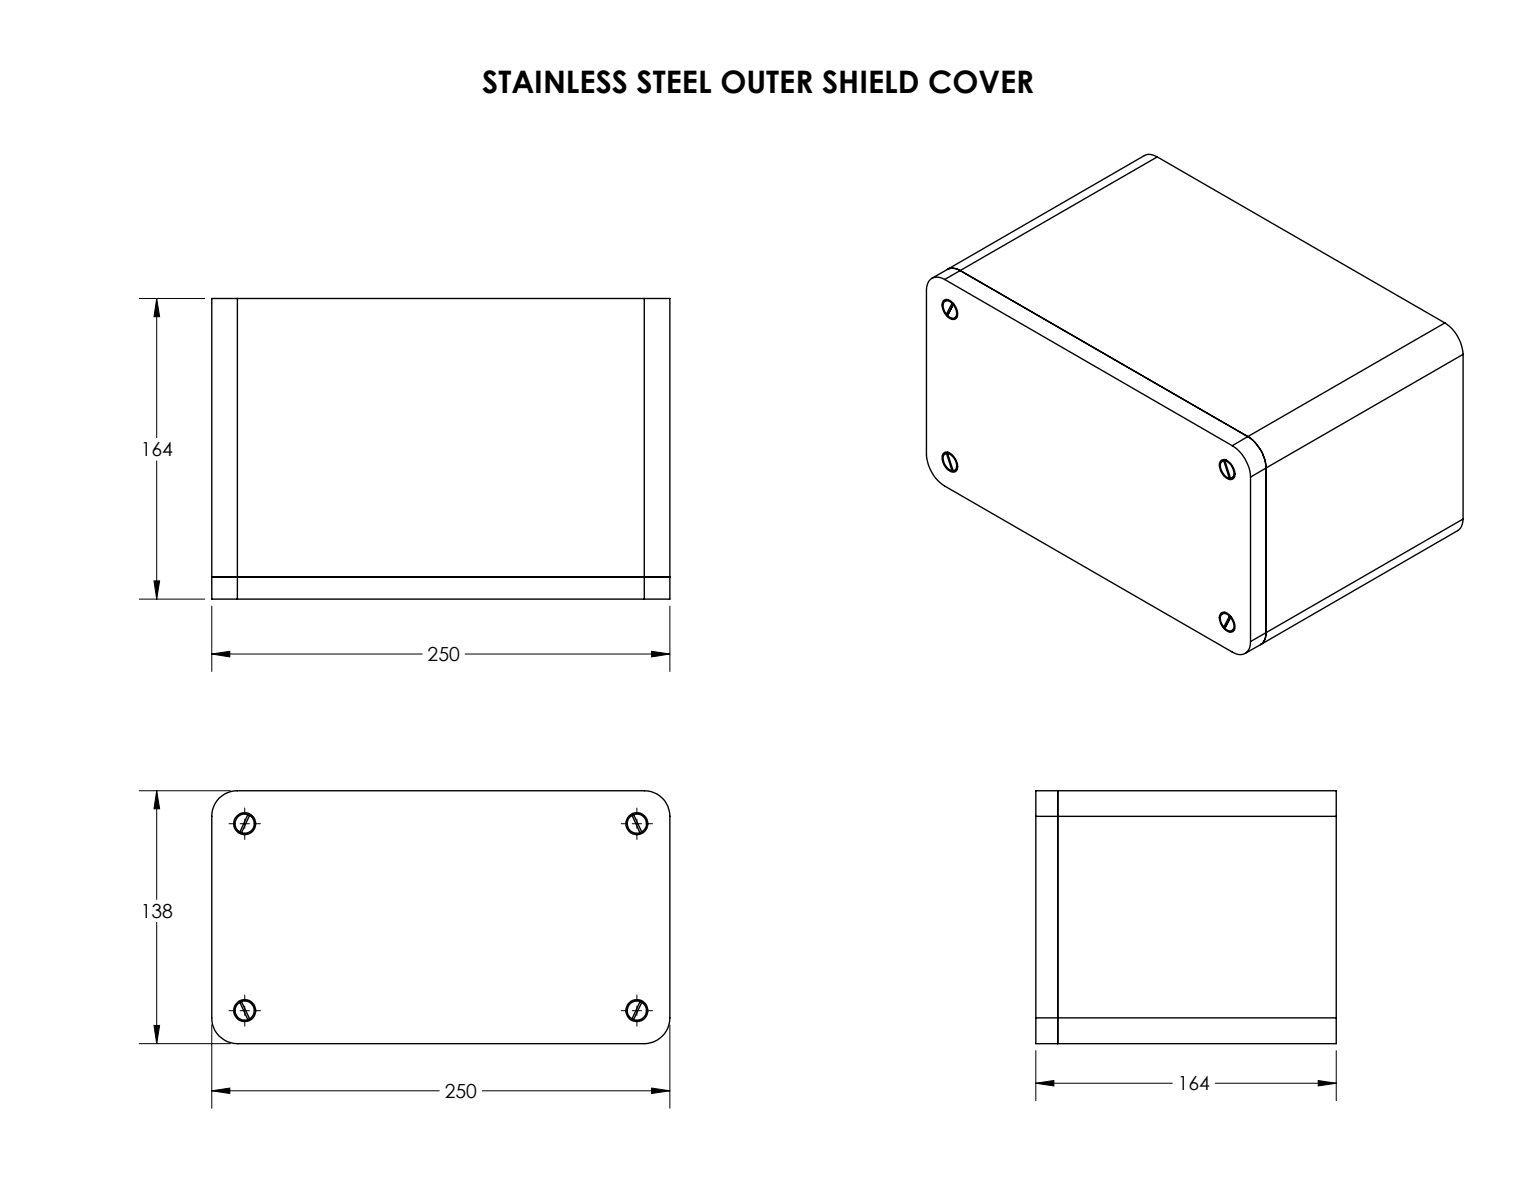
ISO-10303-21;
HEADER;
FILE_DESCRIPTION (('STEP AP214'),
    '1' );
FILE_NAME ('Stainless Steel Outer Shield Cover.step',
    '2026-10-28T18:30:06',
    ( '' ),
    ( '' ),
    'SwSTEP 2.0',
    'SolidWorks 2024',
    '' );
FILE_SCHEMA (( 'AUTOMOTIVE_DESIGN' ));
ENDSEC;

DATA;
#2=ORIENTED_EDGE ( 'NONE', *, *, #5398, .F. ) ;
#4=DIRECTION ( 'NONE',  ( 5.551115123125772841E-17, -1.848892746611743135E-31, -1.000000000000000000 ) ) ;
#6=CARTESIAN_POINT ( 'NONE',  ( -84.02857808274397655, 98.45434506795682239, 152.0000000000000853 ) ) ;
#9=ORIENTED_EDGE ( 'NONE', *, *, #3496, .F. ) ;
#10=DIRECTION ( 'NONE',  ( 0.4205749795070160557, -0.9072577839912276954, -5.551115123125780853E-17 ) ) ;
#13=EDGE_CURVE ( 'NONE', #832, #1072, #4200, .T. ) ;
#15=VECTOR ( 'NONE', #512, 1000.000000000000000 ) ;
#21=VECTOR ( 'NONE', #4832, 999.9999999999998863 ) ;
#23=CARTESIAN_POINT ( 'NONE',  ( -84.02857808274400497, -39.54565493204319182, -5.551115123125782702E-14 ) ) ;
#25=AXIS2_PLACEMENT_3D ( 'NONE', #1773, #1368, #5093 ) ;
#27=DIRECTION ( 'NONE',  ( -1.000000000000000000, 0.000000000000000000, -7.228014483236656373E-17 ) ) ;
#33=DIRECTION ( 'NONE',  ( 1.000000000000000000, 0.000000000000000000, 0.000000000000000000 ) ) ;
#41=DIRECTION ( 'NONE',  ( -1.000000000000000000, 0.000000000000000000, 0.000000000000000000 ) ) ;
#46=CYLINDRICAL_SURFACE ( 'NONE', #25, 6.000000000000032863 ) ;
#50=CARTESIAN_POINT ( 'NONE',  ( -74.77857808274409024, -21.54565493204320248, -26.84924240491759662 ) ) ;
#51=ORIENTED_EDGE ( 'NONE', *, *, #5105, .T. ) ;
#52=ORIENTED_EDGE ( 'NONE', *, *, #5333, .F. ) ;
#56=EDGE_CURVE ( 'NONE', #1665, #3075, #3058, .T. ) ;
#58=ORIENTED_EDGE ( 'NONE', *, *, #3746, .T. ) ;
#59=PLANE ( 'NONE',  #568 ) ;
#61=EDGE_CURVE ( 'NONE', #167, #979, #3936, .T. ) ;
#62=CARTESIAN_POINT ( 'NONE',  ( -84.02857808274400497, -39.54565493204319893, -11.99999999999984368 ) ) ;
#65=DIRECTION ( 'NONE',  ( -1.000000000000000000, 0.000000000000000000, 0.000000000000000000 ) ) ;
#66=CARTESIAN_POINT ( 'NONE',  ( 133.9714219172562366, -21.54565493204323090, -9.999999999999841904 ) ) ;
#67=ORIENTED_EDGE ( 'NONE', *, *, #2103, .T. ) ;
#72=CARTESIAN_POINT ( 'NONE',  ( -84.02857808274397655, 98.45434506795682239, 152.0000000000000853 ) ) ;
#73=CARTESIAN_POINT ( 'NONE',  ( -98.02857808274420393, -25.54565493204307813, 152.0000000000001990 ) ) ;
#77=CARTESIAN_POINT ( 'NONE',  ( -84.02857808274407603, 84.45434506795682239, -11.99999999999995559 ) ) ;
#79=ORIENTED_EDGE ( 'NONE', *, *, #2485, .T. ) ;
#86=PLANE ( 'NONE',  #1169 ) ;
#89=CARTESIAN_POINT ( 'NONE',  ( 151.9714219172562935, -25.54565493204309234, -5.551115123125782702E-14 ) ) ;
#96=DIRECTION ( 'NONE',  ( 5.551115123125772841E-17, -1.848892746611743135E-31, -1.000000000000000000 ) ) ;
#99=FACE_OUTER_BOUND ( 'NONE', #532, .T. ) ;
#103=ORIENTED_EDGE ( 'NONE', *, *, #5162, .T. ) ;
#106=LINE ( 'NONE', #1784, #5082 ) ;
#107=( NAMED_UNIT ( * ) PLANE_ANGLE_UNIT ( ) SI_UNIT ( $, .RADIAN. ) );
#108=AXIS2_PLACEMENT_3D ( 'NONE', #5417, #1651, #2776 ) ;
#109=EDGE_LOOP ( 'NONE', ( #1428, #2018, #1351, #4648 ) ) ;
#112=DIRECTION ( 'NONE',  ( 5.551115123125772841E-17, -1.848892746611743135E-31, -1.000000000000000000 ) ) ;
#116=CARTESIAN_POINT ( 'NONE',  ( 127.9714219172562224, -21.54565493204319182, -2.000000000000002220 ) ) ;
#118=ORIENTED_EDGE ( 'NONE', *, *, #13, .F. ) ;
#122=LINE ( 'NONE', #1849, #2478 ) ;
#125=AXIS2_PLACEMENT_3D ( 'NONE', #1233, #2528, #573 ) ;
#126=AXIS2_PLACEMENT_3D ( 'NONE', #266, #1941, #351 ) ;
#128=ORIENTED_EDGE ( 'NONE', *, *, #2251, .T. ) ;
#131=AXIS2_PLACEMENT_3D ( 'NONE', #4848, #2356, #4561 ) ;
#132=AXIS2_PLACEMENT_3D ( 'NONE', #1581, #2880, #843 ) ;
#133=CARTESIAN_POINT ( 'NONE',  ( 136.6230329513293213, 75.92317977368846016, -10.00000000000006395 ) ) ;
#135=CARTESIAN_POINT ( 'NONE',  ( -77.37696704867106234, 84.98551036222526989, -9.999999999999953815 ) ) ;
#141=EDGE_LOOP ( 'NONE', ( #309, #4866, #1878, #776 ) ) ;
#143=DIRECTION ( 'NONE',  ( -5.551115123125772841E-17, 1.848892746611743135E-31, 1.000000000000000000 ) ) ;
#145=DIRECTION ( 'NONE',  ( 5.551115123125772841E-17, -1.848892746611743135E-31, -1.000000000000000000 ) ) ;
#146=ORIENTED_EDGE ( 'NONE', *, *, #3858, .T. ) ;
#150=CARTESIAN_POINT ( 'NONE',  ( 132.2270686671744500, 85.40608534173220789, -11.99999999999990052 ) ) ;
#167=VERTEX_POINT ( 'NONE', #1947 ) ;
#170=CARTESIAN_POINT ( 'NONE',  ( -84.02857808274403340, 98.45434506795682239, -12.00000000000001066 ) ) ;
#177=CARTESIAN_POINT ( 'NONE',  ( 135.7157751673380801, 75.50260479418143689, -10.00000000000006395 ) ) ;
#179=VERTEX_POINT ( 'NONE', #3708 ) ;
#182=DIRECTION ( 'NONE',  ( 5.551115123125772841E-17, -1.848892746611743135E-31, -1.000000000000000000 ) ) ;
#192=CYLINDRICAL_SURFACE ( 'NONE', #816, 5.250000000000018652 ) ;
#200=CARTESIAN_POINT ( 'NONE',  ( -98.02857808274411866, 84.45434506795672291, -12.00000000000001066 ) ) ;
#204=VECTOR ( 'NONE', #2350, 1000.000000000000000 ) ;
#206=ORIENTED_EDGE ( 'NONE', *, *, #2251, .F. ) ;
#207=AXIS2_PLACEMENT_3D ( 'NONE', #2875, #1242, #4553 ) ;
#211=DIRECTION ( 'NONE',  ( 5.551115123125772841E-17, -1.848892746611743135E-31, -1.000000000000000000 ) ) ;
#212=DIRECTION ( 'NONE',  ( -1.000000000000000000, 0.000000000000000000, -7.228014483236656373E-17 ) ) ;
#213=VECTOR ( 'NONE', #927, 1000.000000000000000 ) ;
#215=ORIENTED_EDGE ( 'NONE', *, *, #4294, .F. ) ;
#219=CIRCLE ( 'NONE', #2497, 5.250000000000004441 ) ;
#221=ORIENTED_EDGE ( 'NONE', *, *, #3158, .F. ) ;
#227=ADVANCED_FACE ( 'NONE', ( #4014 ), #4039, .F. ) ;
#230=ADVANCED_FACE ( 'NONE', ( #2825 ), #5293, .T. ) ;
#231=ORIENTED_EDGE ( 'NONE', *, *, #3564, .F. ) ;
#232=CARTESIAN_POINT ( 'NONE',  ( -86.02857808274406182, 80.45434506795689344, -2.000000000000113243 ) ) ;
#234=CARTESIAN_POINT ( 'NONE',  ( -84.02857808274418971, -25.54565493204318116, -5.551115123125782702E-14 ) ) ;
#235=ADVANCED_FACE ( 'NONE', ( #2885 ), #270, .T. ) ;
#238=ORIENTED_EDGE ( 'NONE', *, *, #993, .F. ) ;
#239=CYLINDRICAL_SURFACE ( 'NONE', #132, 5.250000000000004441 ) ;
#241=LINE ( 'NONE', #3933, #1979 ) ;
#242=DIRECTION ( 'NONE',  ( 5.551115123125772841E-17, -1.848892746611743135E-31, -1.000000000000000000 ) ) ;
#244=EDGE_CURVE ( 'NONE', #774, #4710, #3337, .T. ) ;
#252=AXIS2_PLACEMENT_3D ( 'NONE', #1617, #736, #303 ) ;
#254=DIRECTION ( 'NONE',  ( 5.551115123125772841E-17, -1.848892746611743135E-31, -1.000000000000000000 ) ) ;
#258=ADVANCED_FACE ( 'NONE', ( #3277, #1121 ), #4970, .T. ) ;
#259=EDGE_LOOP ( 'NONE', ( #3861, #904 ) ) ;
#260=LINE ( 'NONE', #2757, #3717 ) ;
#261=CARTESIAN_POINT ( 'NONE',  ( 137.9714219172561798, 98.45434506795687923, -5.551115123125782702E-14 ) ) ;
#263=DIRECTION ( 'NONE',  ( 1.000000000000000000, 1.261617073437686134E-16, 5.551115123125772841E-17 ) ) ;
#265=VERTEX_POINT ( 'NONE', #762 ) ;
#266=CARTESIAN_POINT ( 'NONE',  ( -84.02857808274407603, -25.54565493204318116, 152.0000000000000853 ) ) ;
#270=PLANE ( 'NONE',  #773 ) ;
#284=CARTESIAN_POINT ( 'NONE',  ( 133.9714219172562366, 80.45434506795683660, -12.00000000000001066 ) ) ;
#287=PLANE ( 'NONE',  #5276 ) ;
#290=EDGE_LOOP ( 'NONE', ( #3671, #3262, #5267, #5005 ) ) ;
#293=AXIS2_PLACEMENT_3D ( 'NONE', #771, #797, #2891 ) ;
#296=LINE ( 'NONE', #4968, #4867 ) ;
#297=AXIS2_PLACEMENT_3D ( 'NONE', #1076, #5275, #777 ) ;
#299=CARTESIAN_POINT ( 'NONE',  ( 137.9714219172563219, 84.45434506795683660, 152.0000000000003126 ) ) ;
#301=CIRCLE ( 'NONE', #3552, 14.00000000000002665 ) ;
#303=DIRECTION ( 'NONE',  ( 1.000000000000000000, 0.000000000000000000, 0.000000000000000000 ) ) ;
#308=AXIS2_PLACEMENT_3D ( 'NONE', #4986, #4222, #450 ) ;
#309=ORIENTED_EDGE ( 'NONE', *, *, #61, .T. ) ;
#311=PRODUCT_DEFINITION_SHAPE ( 'NONE', 'NONE',  #377 ) ;
#312=ORIENTED_EDGE ( 'NONE', *, *, #5219, .T. ) ;
#315=ORIENTED_EDGE ( 'NONE', *, *, #1838, .F. ) ;
#317=CARTESIAN_POINT ( 'NONE',  ( 132.2270686671743931, -26.49739520581860219, -11.99999999999990052 ) ) ;
#329=DIRECTION ( 'NONE',  ( -1.000000000000000000, 3.759415251443877379E-31, -5.551115123125772841E-17 ) ) ;
#339=VERTEX_POINT ( 'NONE', #1718 ) ;
#340=AXIS2_PLACEMENT_3D ( 'NONE', #1650, #345, #2021 ) ;
#345=DIRECTION ( 'NONE',  ( 5.551115123125772841E-17, -1.848892746611743354E-31, -1.000000000000000000 ) ) ;
#347=CYLINDRICAL_SURFACE ( 'NONE', #2595, 5.250000000000004441 ) ;
#348=DIRECTION ( 'NONE',  ( -1.000000000000000000, 0.000000000000000000, -7.228014483236656373E-17 ) ) ;
#351=DIRECTION ( 'NONE',  ( 1.000000000000000000, 0.000000000000000000, 0.000000000000000000 ) ) ;
#359=ORIENTED_EDGE ( 'NONE', *, *, #3631, .F. ) ;
#363=VECTOR ( 'NONE', #4645, 1000.000000000000000 ) ;
#364=CARTESIAN_POINT ( 'NONE',  ( -74.02857808274400497, 80.45434506795689344, -12.00000000000001066 ) ) ;
#369=DIRECTION ( 'NONE',  ( 5.551115123125772841E-17, -1.848892746611743135E-31, -1.000000000000000000 ) ) ;
#372=VECTOR ( 'NONE', #375, 1000.000000000000114 ) ;
#373=EDGE_LOOP ( 'NONE', ( #2567, #146 ) ) ;
#375=DIRECTION ( 'NONE',  ( -0.4205749795070158337, -0.9072577839912276954, 0.000000000000000000 ) ) ;
#377=PRODUCT_DEFINITION ( 'UNKNOWN', '', #3741, #713 ) ;
#380=AXIS2_PLACEMENT_3D ( 'NONE', #3630, #3981, #212 ) ;
#382=VECTOR ( 'NONE', #4088, 1000.000000000000000 ) ;
#387=ORIENTED_EDGE ( 'NONE', *, *, #567, .T. ) ;
#388=CARTESIAN_POINT ( 'NONE',  ( -84.02857808274400497, -39.54565493204319182, -5.551115123125782702E-14 ) ) ;
#389=VECTOR ( 'NONE', #3370, 1000.000000000000000 ) ;
#393=ORIENTED_EDGE ( 'NONE', *, *, #490, .T. ) ;
#396=ADVANCED_FACE ( 'NONE', ( #2658 ), #3931, .F. ) ;
#405=VERTEX_POINT ( 'NONE', #133 ) ;
#406=EDGE_LOOP ( 'NONE', ( #3376, #2068, #1234, #4289 ) ) ;
#412=DIRECTION ( 'NONE',  ( -0.4205749795070160002, 0.9072577839912275843, 5.551115123125780237E-17 ) ) ;
#413=ORIENTED_EDGE ( 'NONE', *, *, #3394, .T. ) ;
#417=ORIENTED_EDGE ( 'NONE', *, *, #5228, .F. ) ;
#421=CARTESIAN_POINT ( 'NONE',  ( -84.02857808274407603, -25.54565493204318116, 152.0000000000000853 ) ) ;
#422=EDGE_CURVE ( 'NONE', #850, #3905, #3161, .T. ) ;
#428=DIRECTION ( 'NONE',  ( 5.551115123125772841E-17, -1.848892746611743135E-31, -1.000000000000000000 ) ) ;
#434=CARTESIAN_POINT ( 'NONE',  ( 151.9714219172563219, 84.45434506795673713, 152.0000000000001990 ) ) ;
#435=ORIENTED_EDGE ( 'NONE', *, *, #5189, .F. ) ;
#439=ORIENTED_EDGE ( 'NONE', *, *, #3868, .F. ) ;
#440=CARTESIAN_POINT ( 'NONE',  ( 151.9714219172562935, -25.54565493204307813, 152.0000000000001990 ) ) ;
#444=PLANE ( 'NONE',  #340 ) ;
#447=EDGE_LOOP ( 'NONE', ( #103, #5217, #5036, #2948 ) ) ;
#450=DIRECTION ( 'NONE',  ( 1.000000000000000000, -3.759415251443877379E-31, 5.551115123125772841E-17 ) ) ;
#451=CARTESIAN_POINT ( 'NONE',  ( 137.9714219172561513, -25.54565493204318116, -11.99999999999995559 ) ) ;
#453=LINE ( 'NONE', #2135, #4250 ) ;
#455=CIRCLE ( 'NONE', #1157, 5.250000000000018652 ) ;
#461=ADVANCED_FACE ( 'NONE', ( #99 ), #4338, .F. ) ;
#465=VECTOR ( 'NONE', #4114, 1000.000000000000114 ) ;
#466=CIRCLE ( 'NONE', #293, 6.000000000000032863 ) ;
#467=VERTEX_POINT ( 'NONE', #1777 ) ;
#468=DIRECTION ( 'NONE',  ( -1.000000000000000000, 0.000000000000000000, -5.551115123125777155E-17 ) ) ;
#471=CIRCLE ( 'NONE', #1001, 14.00000000000002665 ) ;
#473=DIRECTION ( 'NONE',  ( 5.551115123125772841E-17, -1.848892746611743135E-31, -1.000000000000000000 ) ) ;
#483=VERTEX_POINT ( 'NONE', #931 ) ;
#484=VERTEX_POINT ( 'NONE', #4388 ) ;
#486=VERTEX_POINT ( 'NONE', #4365 ) ;
#490=EDGE_CURVE ( 'NONE', #2425, #3390, #3076, .T. ) ;
#491=DIRECTION ( 'NONE',  ( -5.551115123125772841E-17, 1.848892746611743354E-31, 1.000000000000000000 ) ) ;
#495=DIRECTION ( 'NONE',  ( -1.000000000000000000, 0.000000000000000000, 0.000000000000000000 ) ) ;
#496=VERTEX_POINT ( 'NONE', #3951 ) ;
#499=EDGE_CURVE ( 'NONE', #3639, #1984, #944, .T. ) ;
#502=CARTESIAN_POINT ( 'NONE',  ( -80.02857808274410445, -21.54565493204320248, -12.00000000000001066 ) ) ;
#505=DIRECTION ( 'NONE',  ( 5.551115123125772841E-17, -1.848892746611743135E-31, -1.000000000000000000 ) ) ;
#508=ORIENTED_EDGE ( 'NONE', *, *, #1839, .F. ) ;
#509=VECTOR ( 'NONE', #1316, 1000.000000000000000 ) ;
#510=ORIENTED_EDGE ( 'NONE', *, *, #2344, .T. ) ;
#512=DIRECTION ( 'NONE',  ( 1.261617073437686134E-16, -1.000000000000000000, -1.232595164407830946E-31 ) ) ;
#518=PLANE ( 'NONE',  #2144 ) ;
#520=ORIENTED_EDGE ( 'NONE', *, *, #1534, .F. ) ;
#531=EDGE_CURVE ( 'NONE', #2111, #5400, #1371, .T. ) ;
#532=EDGE_LOOP ( 'NONE', ( #58, #3431, #3991, #3373 ) ) ;
#534=VERTEX_POINT ( 'NONE', #954 ) ;
#544=VECTOR ( 'NONE', #3570, 1000.000000000000000 ) ;
#552=EDGE_LOOP ( 'NONE', ( #2201, #2575, #4436, #4481 ) ) ;
#555=CARTESIAN_POINT ( 'NONE',  ( 131.3198108831832087, -26.07682022631159668, -10.00000000000000888 ) ) ;
#556=VERTEX_POINT ( 'NONE', #4820 ) ;
#565=CARTESIAN_POINT ( 'NONE',  ( 133.9714219172562366, -21.54565493204319182, -12.00000000000006573 ) ) ;
#567=EDGE_CURVE ( 'NONE', #5400, #5147, #758, .T. ) ;
#568=AXIS2_PLACEMENT_3D ( 'NONE', #4963, #3656, #5315 ) ;
#569=ORIENTED_EDGE ( 'NONE', *, *, #531, .T. ) ;
#571=DIRECTION ( 'NONE',  ( 1.000000000000000000, -3.759415251443877817E-31, 5.551115123125772841E-17 ) ) ;
#573=DIRECTION ( 'NONE',  ( 1.000000000000000000, 0.000000000000000000, 0.000000000000000000 ) ) ;
#574=( GEOMETRIC_REPRESENTATION_CONTEXT ( 3 ) GLOBAL_UNCERTAINTY_ASSIGNED_CONTEXT ( ( #3923 ) ) GLOBAL_UNIT_ASSIGNED_CONTEXT ( ( #5102, #107, #4619 ) ) REPRESENTATION_CONTEXT ( 'NONE', 'WORKASPACE' ) );
#577=VERTEX_POINT ( 'NONE', #5347 ) ;
#579=ORIENTED_EDGE ( 'NONE', *, *, #2512, .T. ) ;
#580=DIRECTION ( 'NONE',  ( -1.000000000000000000, 0.000000000000000000, 0.000000000000000000 ) ) ;
#585=ADVANCED_FACE ( 'NONE', ( #1973 ), #4098, .F. ) ;
#593=CARTESIAN_POINT ( 'NONE',  ( -80.02857808274401918, 80.45434506795689344, -2.000000000000112799 ) ) ;
#595=DIRECTION ( 'NONE',  ( 5.551115123125772841E-17, -1.848892746611743135E-31, -1.000000000000000000 ) ) ;
#605=EDGE_LOOP ( 'NONE', ( #4984, #2778, #4803, #4779 ) ) ;
#609=CARTESIAN_POINT ( 'NONE',  ( -80.02857808274401918, 80.45434506795689344, -2.000000000000112799 ) ) ;
#611=EDGE_LOOP ( 'NONE', ( #3586, #3264, #2074, #924 ) ) ;
#617=EDGE_CURVE ( 'NONE', #3157, #2425, #2058, .T. ) ;
#618=EDGE_CURVE ( 'NONE', #2650, #994, #2027, .T. ) ;
#619=DIRECTION ( 'NONE',  ( 1.000000000000000000, 0.000000000000000000, 5.551115123125771609E-17 ) ) ;
#624=ADVANCED_FACE ( 'NONE', ( #4473 ), #4879, .F. ) ;
#627=ORIENTED_EDGE ( 'NONE', *, *, #3002, .F. ) ;
#630=CARTESIAN_POINT ( 'NONE',  ( -77.37696704867106234, 84.98551036222526989, -9.999999999999953815 ) ) ;
#638=FACE_BOUND ( 'NONE', #3051, .T. ) ;
#641=AXIS2_PLACEMENT_3D ( 'NONE', #2055, #3740, #4584 ) ;
#644=EDGE_CURVE ( 'NONE', #2687, #4195, #1144, .T. ) ;
#645=FACE_OUTER_BOUND ( 'NONE', #5047, .T. ) ;
#650=CARTESIAN_POINT ( 'NONE',  ( 137.9714219172562082, 98.45434506795683660, 152.0000000000003126 ) ) ;
#651=FACE_OUTER_BOUND ( 'NONE', #1633, .T. ) ;
#653=AXIS2_PLACEMENT_3D ( 'NONE', #3593, #2347, #4054 ) ;
#654=ORIENTED_EDGE ( 'NONE', *, *, #4717, .T. ) ;
#658=ADVANCED_FACE ( 'NONE', ( #2822 ), #2354, .T. ) ;
#662=DIRECTION ( 'NONE',  ( 5.551115123125772841E-17, -1.848892746611743135E-31, -1.000000000000000000 ) ) ;
#664=VERTEX_POINT ( 'NONE', #4035 ) ;
#667=CARTESIAN_POINT ( 'NONE',  ( -85.27857808274403340, 80.45434506795689344, -2.000000000000113243 ) ) ;
#669=LINE ( 'NONE', #3700, #1684 ) ;
#670=DIRECTION ( 'NONE',  ( 5.551115123125772841E-17, -1.848892746611743135E-31, -1.000000000000000000 ) ) ;
#671=ORIENTED_EDGE ( 'NONE', *, *, #3189, .F. ) ;
#672=DIRECTION ( 'NONE',  ( 5.551115123125772841E-17, -1.848892746611743135E-31, -1.000000000000000000 ) ) ;
#681=ADVANCED_FACE ( 'NONE', ( #2326 ), #239, .T. ) ;
#686=PLANE ( 'NONE',  #989 ) ;
#688=ORIENTED_EDGE ( 'NONE', *, *, #4703, .T. ) ;
#698=DIRECTION ( 'NONE',  ( 5.551115123125772841E-17, -1.848892746611743135E-31, -1.000000000000000000 ) ) ;
#710=LINE ( 'NONE', #630, #2231 ) ;
#711=AXIS2_PLACEMENT_3D ( 'NONE', #1713, #2130, #4280 ) ;
#713=PRODUCT_DEFINITION_CONTEXT ( 'detailed design', #2438, 'design' ) ;
#716=DIRECTION ( 'NONE',  ( -1.000000000000000000, 0.000000000000000000, -7.228014483236656373E-17 ) ) ;
#720=EDGE_CURVE ( 'NONE', #1930, #1984, #2928, .T. ) ;
#721=CARTESIAN_POINT ( 'NONE',  ( 151.9714219172563219, 84.45434506795673713, 152.0000000000001990 ) ) ;
#723=VECTOR ( 'NONE', #4325, 1000.000000000000000 ) ;
#729=LINE ( 'NONE', #5348, #1860 ) ;
#730=CARTESIAN_POINT ( 'NONE',  ( -84.02857808274407603, 84.45434506795682239, -11.99999999999995559 ) ) ;
#736=DIRECTION ( 'NONE',  ( -5.551115123125772841E-17, 1.848892746611743135E-31, 1.000000000000000000 ) ) ;
#739=CIRCLE ( 'NONE', #5297, 5.250000000000004441 ) ;
#747=ORIENTED_EDGE ( 'NONE', *, *, #3002, .T. ) ;
#749=DIRECTION ( 'NONE',  ( -1.000000000000000000, 0.000000000000000000, -5.551115123125777155E-17 ) ) ;
#750=CARTESIAN_POINT ( 'NONE',  ( 139.2214219172562366, -21.54565493204319182, -2.000000000000001332 ) ) ;
#755=ORIENTED_EDGE ( 'NONE', *, *, #3729, .T. ) ;
#758=LINE ( 'NONE', #2382, #5292 ) ;
#762=CARTESIAN_POINT ( 'NONE',  ( -74.77857808274401918, 80.45434506795689344, -12.00000000000001066 ) ) ;
#770=VECTOR ( 'NONE', #1379, 1000.000000000000000 ) ;
#771=CARTESIAN_POINT ( 'NONE',  ( -80.02857808274410445, -21.54565493204320248, -12.00000000000001066 ) ) ;
#772=DIRECTION ( 'NONE',  ( -5.551115123125772841E-17, 1.848892746611743135E-31, 1.000000000000000000 ) ) ;
#773=AXIS2_PLACEMENT_3D ( 'NONE', #3310, #5322, #2422 ) ;
#774=VERTEX_POINT ( 'NONE', #4607 ) ;
#776=ORIENTED_EDGE ( 'NONE', *, *, #4366, .T. ) ;
#777=DIRECTION ( 'NONE',  ( 1.000000000000000000, 0.000000000000000000, 7.228014483236656373E-17 ) ) ;
#780=CARTESIAN_POINT ( 'NONE',  ( 151.9714219172562935, -25.54565493204307813, 152.0000000000001990 ) ) ;
#782=ORIENTED_EDGE ( 'NONE', *, *, #3083, .F. ) ;
#783=VERTEX_POINT ( 'NONE', #3735 ) ;
#788=FACE_OUTER_BOUND ( 'NONE', #2745, .T. ) ;
#793=EDGE_LOOP ( 'NONE', ( #1954, #4146, #1989, #3668, #231, #2566, #1032, #3056 ) ) ;
#795=EDGE_CURVE ( 'NONE', #265, #3229, #3649, .T. ) ;
#797=DIRECTION ( 'NONE',  ( 5.551115123125772841E-17, -1.848892746611743135E-31, -1.000000000000000000 ) ) ;
#800=VERTEX_POINT ( 'NONE', #865 ) ;
#804=DIRECTION ( 'NONE',  ( 5.551115123125772841E-17, -1.848892746611743354E-31, -1.000000000000000000 ) ) ;
#805=AXIS2_PLACEMENT_3D ( 'NONE', #5064, #4987, #5008 ) ;
#806=ORIENTED_EDGE ( 'NONE', *, *, #5430, .T. ) ;
#808=ORIENTED_EDGE ( 'NONE', *, *, #2585, .T. ) ;
#811=DIRECTION ( 'NONE',  ( 5.551115123125772841E-17, -1.848892746611743135E-31, -1.000000000000000000 ) ) ;
#812=CIRCLE ( 'NONE', #2398, 14.00000000000001243 ) ;
#813=ADVANCED_FACE ( 'NONE', ( #4252, #3350 ), #2545, .F. ) ;
#816=AXIS2_PLACEMENT_3D ( 'NONE', #1900, #4808, #4021 ) ;
#821=VECTOR ( 'NONE', #1526, 1000.000000000000000 ) ;
#827=VECTOR ( 'NONE', #4315, 1000.000000000000000 ) ;
#832=VERTEX_POINT ( 'NONE', #4659 ) ;
#841=ORIENTED_EDGE ( 'NONE', *, *, #3959, .F. ) ;
#843=DIRECTION ( 'NONE',  ( 1.000000000000000000, 0.000000000000000000, 0.000000000000000000 ) ) ;
#846=CARTESIAN_POINT ( 'NONE',  ( 137.9714219172561798, 98.45434506795689344, -5.551115123125782702E-14 ) ) ;
#849=CARTESIAN_POINT ( 'NONE',  ( -74.77857808274410445, -21.54565493204320248, -12.00000000000001066 ) ) ;
#850=VERTEX_POINT ( 'NONE', #891 ) ;
#855=CARTESIAN_POINT ( 'NONE',  ( -78.28422483266226095, 85.40608534173227895, -10.00000000000006395 ) ) ;
#856=LINE ( 'NONE', #1649, #465 ) ;
#857=CARTESIAN_POINT ( 'NONE',  ( -78.28422483266231779, -26.49739520581859153, -10.00000000000006395 ) ) ;
#864=VERTEX_POINT ( 'NONE', #3862 ) ;
#865=CARTESIAN_POINT ( 'NONE',  ( 135.7157751673381370, -16.59391465826787027, -11.99999999999995559 ) ) ;
#866=ADVANCED_FACE ( 'NONE', ( #975 ), #3946, .T. ) ;
#868=CARTESIAN_POINT ( 'NONE',  ( 133.9714219172562366, -21.54565493204319182, -2.000000000000001776 ) ) ;
#874=ORIENTED_EDGE ( 'NONE', *, *, #2540, .F. ) ;
#878=CYLINDRICAL_SURFACE ( 'NONE', #2935, 5.250000000000018652 ) ;
#881=LINE ( 'NONE', #2439, #2057 ) ;
#886=DIRECTION ( 'NONE',  ( 5.551115123125772841E-17, -1.848892746611743135E-31, -1.000000000000000000 ) ) ;
#887=DIRECTION ( 'NONE',  ( -1.000000000000000000, 3.759415251443877379E-31, -5.551115123125772841E-17 ) ) ;
#891=CARTESIAN_POINT ( 'NONE',  ( -98.02857808274411866, 84.45434506795672291, 152.0000000000001990 ) ) ;
#892=DIRECTION ( 'NONE',  ( -1.000000000000000000, 0.000000000000000000, 0.000000000000000000 ) ) ;
#893=CARTESIAN_POINT ( 'NONE',  ( -80.02857808274401918, 80.45434506795689344, -12.00000000000001066 ) ) ;
#904=ORIENTED_EDGE ( 'NONE', *, *, #244, .T. ) ;
#909=CARTESIAN_POINT ( 'NONE',  ( 132.2270686671745068, 85.40608534173219368, -9.999999999999953815 ) ) ;
#912=DIRECTION ( 'NONE',  ( 5.551115123125772841E-17, -1.848892746611743135E-31, -1.000000000000000000 ) ) ;
#918=CARTESIAN_POINT ( 'NONE',  ( 133.9714219172562366, -21.54565493204319182, -12.00000000000006573 ) ) ;
#919=CIRCLE ( 'NONE', #2241, 5.250000000000018652 ) ;
#920=CIRCLE ( 'NONE', #653, 5.250000000000004441 ) ;
#921=VERTEX_POINT ( 'NONE', #5197 ) ;
#924=ORIENTED_EDGE ( 'NONE', *, *, #5184, .F. ) ;
#927=DIRECTION ( 'NONE',  ( 5.551115123125772841E-17, -1.848892746611743135E-31, -1.000000000000000000 ) ) ;
#930=ORIENTED_EDGE ( 'NONE', *, *, #3430, .F. ) ;
#931=CARTESIAN_POINT ( 'NONE',  ( -84.02857808274400497, -39.54565493204319182, -5.551115123125782702E-14 ) ) ;
#933=CARTESIAN_POINT ( 'NONE',  ( -81.77293133282597637, 75.50260479418152215, -10.00000000000000888 ) ) ;
#944=CIRCLE ( 'NONE', #5153, 5.250000000000018652 ) ;
#945=ORIENTED_EDGE ( 'NONE', *, *, #5283, .F. ) ;
#953=AXIS2_PLACEMENT_3D ( 'NONE', #5351, #4856, #4103 ) ;
#954=CARTESIAN_POINT ( 'NONE',  ( -74.02857808274400497, 80.45434506795689344, -2.000000000000112355 ) ) ;
#956=CARTESIAN_POINT ( 'NONE',  ( -80.02857808274401918, 80.45434506795689344, -2.000000000000112799 ) ) ;
#959=DIRECTION ( 'NONE',  ( 0.000000000000000000, 0.000000000000000000, 1.000000000000000000 ) ) ;
#962=ORIENTED_EDGE ( 'NONE', *, *, #4572, .T. ) ;
#964=VERTEX_POINT ( 'NONE', #4383 ) ;
#974=ORIENTED_EDGE ( 'NONE', *, *, #4199, .T. ) ;
#975=FACE_OUTER_BOUND ( 'NONE', #2093, .T. ) ;
#976=CARTESIAN_POINT ( 'NONE',  ( -98.02857808274411866, 84.45434506795672291, 152.0000000000001990 ) ) ;
#979=VERTEX_POINT ( 'NONE', #261 ) ;
#982=CARTESIAN_POINT ( 'NONE',  ( 133.9714219172562650, 80.45434506795682239, -9.999999999999841904 ) ) ;
#985=AXIS2_PLACEMENT_3D ( 'NONE', #2897, #886, #65 ) ;
#986=DIRECTION ( 'NONE',  ( -5.551115123125772841E-17, 1.848892746611743135E-31, 1.000000000000000000 ) ) ;
#989=AXIS2_PLACEMENT_3D ( 'NONE', #1462, #4401, #3145 ) ;
#990=VECTOR ( 'NONE', #1669, 1000.000000000000000 ) ;
#991=ORIENTED_EDGE ( 'NONE', *, *, #1776, .T. ) ;
#993=EDGE_CURVE ( 'NONE', #484, #1678, #920, .T. ) ;
#994=VERTEX_POINT ( 'NONE', #667 ) ;
#996=CIRCLE ( 'NONE', #3207, 6.000000000000032863 ) ;
#1000=ORIENTED_EDGE ( 'NONE', *, *, #1392, .F. ) ;
#1001=AXIS2_PLACEMENT_3D ( 'NONE', #4562, #5404, #2498 ) ;
#1011=MECHANICAL_DESIGN_GEOMETRIC_PRESENTATION_REPRESENTATION('',(#3477),#1358);
#1013=DIRECTION ( 'NONE',  ( 5.551115123125772841E-17, -1.848892746611743135E-31, -1.000000000000000000 ) ) ;
#1022=VECTOR ( 'NONE', #4134, 1000.000000000000114 ) ;
#1023=DIRECTION ( 'NONE',  ( -1.000000000000000000, 2.523234146875361914E-16, -5.551115123125772841E-17 ) ) ;
#1024=ORIENTED_EDGE ( 'NONE', *, *, #4393, .F. ) ;
#1025=EDGE_LOOP ( 'NONE', ( #3853, #1190, #2161 ) ) ;
#1032=ORIENTED_EDGE ( 'NONE', *, *, #4823, .F. ) ;
#1036=EDGE_CURVE ( 'NONE', #4330, #921, #4093, .T. ) ;
#1042=VERTEX_POINT ( 'NONE', #4491 ) ;
#1047=EDGE_LOOP ( 'NONE', ( #5067, #3342 ) ) ;
#1059=CYLINDRICAL_SURFACE ( 'NONE', #3018, 14.00000000000002665 ) ;
#1060=EDGE_CURVE ( 'NONE', #339, #1068, #4635, .T. ) ;
#1066=VERTEX_POINT ( 'NONE', #4004 ) ;
#1068=VERTEX_POINT ( 'NONE', #2376 ) ;
#1070=CARTESIAN_POINT ( 'NONE',  ( -81.77293133282597637, 75.50260479418152215, -10.00000000000000888 ) ) ;
#1071=VECTOR ( 'NONE', #4116, 1000.000000000000000 ) ;
#1072=VERTEX_POINT ( 'NONE', #750 ) ;
#1076=CARTESIAN_POINT ( 'NONE',  ( -80.02857808274401918, 80.45434506795689344, -2.000000000000112799 ) ) ;
#1078=DIRECTION ( 'NONE',  ( -5.551115123125772841E-17, 1.848892746611743135E-31, 1.000000000000000000 ) ) ;
#1080=MECHANICAL_DESIGN_GEOMETRIC_PRESENTATION_REPRESENTATION('',(#2751),#1786);
#1083=EDGE_CURVE ( 'NONE', #4995, #4404, #1489, .T. ) ;
#1086=CARTESIAN_POINT ( 'NONE',  ( -78.28422483266231779, -26.49739520581859153, -10.00000000000006395 ) ) ;
#1087=CIRCLE ( 'NONE', #4172, 6.000000000000032863 ) ;
#1091=CARTESIAN_POINT ( 'NONE',  ( 136.6230329513293213, 75.92317977368846016, -10.00000000000006395 ) ) ;
#1092=AXIS2_PLACEMENT_3D ( 'NONE', #3410, #5065, #1307 ) ;
#1097=LINE ( 'NONE', #3451, #3193 ) ;
#1098=ORIENTED_EDGE ( 'NONE', *, *, #244, .F. ) ;
#1100=ORIENTED_EDGE ( 'NONE', *, *, #1377, .T. ) ;
#1104=DIRECTION ( 'NONE',  ( 5.551115123125772841E-17, -1.848892746611743135E-31, -1.000000000000000000 ) ) ;
#1110=CARTESIAN_POINT ( 'NONE',  ( 133.9714219172562366, -21.54565493204319182, -12.00000000000006573 ) ) ;
#1112=DIRECTION ( 'NONE',  ( -5.551115123125772841E-17, 1.848892746611743135E-31, 1.000000000000000000 ) ) ;
#1113=ORIENTED_EDGE ( 'NONE', *, *, #1498, .T. ) ;
#1116=DIRECTION ( 'NONE',  ( 0.4205749795070160002, -0.9072577839912275843, -5.551115123125780237E-17 ) ) ;
#1118=CARTESIAN_POINT ( 'NONE',  ( 131.3198108831832371, 84.98551036222518462, -11.99999999999995559 ) ) ;
#1121=FACE_OUTER_BOUND ( 'NONE', #5169, .T. ) ;
#1128=EDGE_LOOP ( 'NONE', ( #79, #4658, #3456, #2909 ) ) ;
#1131=ADVANCED_FACE ( 'NONE', ( #638, #2318, #1905, #2758, #1219 ), #444, .T. ) ;
#1134=ADVANCED_FACE ( 'NONE', ( #1629 ), #3319, .F. ) ;
#1140=DIRECTION ( 'NONE',  ( 5.551115123125772841E-17, -1.848892746611743135E-31, -1.000000000000000000 ) ) ;
#1144=LINE ( 'NONE', #2853, #3382 ) ;
#1154=DIRECTION ( 'NONE',  ( -1.000000000000000000, 0.000000000000000000, -5.551115123125777155E-17 ) ) ;
#1157=AXIS2_PLACEMENT_3D ( 'NONE', #2494, #428, #3777 ) ;
#1160=VERTEX_POINT ( 'NONE', #4550 ) ;
#1165=FACE_OUTER_BOUND ( 'NONE', #5126, .T. ) ;
#1166=FACE_OUTER_BOUND ( 'NONE', #2458, .T. ) ;
#1169=AXIS2_PLACEMENT_3D ( 'NONE', #3003, #2596, #4711 ) ;
#1176=VECTOR ( 'NONE', #2186, 1000.000000000000000 ) ;
#1177=VECTOR ( 'NONE', #1492, 1000.000000000000000 ) ;
#1178=DIRECTION ( 'NONE',  ( 5.551115123125772841E-17, -1.848892746611743354E-31, -1.000000000000000000 ) ) ;
#1184=ORIENTED_EDGE ( 'NONE', *, *, #5158, .F. ) ;
#1190=ORIENTED_EDGE ( 'NONE', *, *, #4135, .T. ) ;
#1194=CARTESIAN_POINT ( 'NONE',  ( -86.02857808274421814, -21.54565493204321669, -2.000000000000002220 ) ) ;
#1196=CARTESIAN_POINT ( 'NONE',  ( 137.9714219172561229, -39.54565493204319182, 152.0000000000004263 ) ) ;
#1197=ORIENTED_EDGE ( 'NONE', *, *, #4921, .T. ) ;
#1200=CARTESIAN_POINT ( 'NONE',  ( -77.37696704867111919, -26.07682022631158247, -11.99999999999995559 ) ) ;
#1205=CARTESIAN_POINT ( 'NONE',  ( 127.9714219172562508, 80.45434506795683660, -2.000000000000002220 ) ) ;
#1211=EDGE_CURVE ( 'NONE', #2228, #4995, #4980, .T. ) ;
#1218=CARTESIAN_POINT ( 'NONE',  ( -80.02857808274401918, 80.45434506795689344, -2.000000000000112799 ) ) ;
#1219=FACE_OUTER_BOUND ( 'NONE', #3407, .T. ) ;
#1222=DIRECTION ( 'NONE',  ( 0.4205749795070160002, -0.9072577839912275843, -5.551115123125780237E-17 ) ) ;
#1224=ORIENTED_EDGE ( 'NONE', *, *, #4717, .F. ) ;
#1233=CARTESIAN_POINT ( 'NONE',  ( 133.9714219172562650, 80.45434506795682239, -9.999999999999841904 ) ) ;
#1234=ORIENTED_EDGE ( 'NONE', *, *, #2105, .F. ) ;
#1242=DIRECTION ( 'NONE',  ( 5.551115123125772841E-17, -1.848892746611743135E-31, -1.000000000000000000 ) ) ;
#1245=AXIS2_PLACEMENT_3D ( 'NONE', #3918, #3091, #1950 ) ;
#1248=CARTESIAN_POINT ( 'NONE',  ( 151.9714219172563219, 84.45434506795677976, -5.551115123125782702E-14 ) ) ;
#1252=AXIS2_PLACEMENT_3D ( 'NONE', #4037, #5290, #4418 ) ;
#1254=VECTOR ( 'NONE', #3150, 1000.000000000000000 ) ;
#1257=AXIS2_PLACEMENT_3D ( 'NONE', #3286, #5022, #4211 ) ;
#1259=ORIENTED_EDGE ( 'NONE', *, *, #2015, .F. ) ;
#1260=CARTESIAN_POINT ( 'NONE',  ( 128.7214219172562650, 80.45434506795679397, -2.000000000000002220 ) ) ;
#1262=AXIS2_PLACEMENT_3D ( 'NONE', #1606, #2117, #27 ) ;
#1265=ORIENTED_EDGE ( 'NONE', *, *, #3424, .T. ) ;
#1269=CARTESIAN_POINT ( 'NONE',  ( 132.2270686671743647, -26.49739520581860219, -9.999999999999953815 ) ) ;
#1271=DIRECTION ( 'NONE',  ( -1.000000000000000000, 0.000000000000000000, 0.000000000000000000 ) ) ;
#1274=ORIENTED_EDGE ( 'NONE', *, *, #56, .F. ) ;
#1276=ORIENTED_EDGE ( 'NONE', *, *, #4199, .F. ) ;
#1277=DIRECTION ( 'NONE',  ( 5.551115123125772841E-17, -1.848892746611743135E-31, -1.000000000000000000 ) ) ;
#1278=DIRECTION ( 'NONE',  ( -5.551115123125772841E-17, 1.848892746611743135E-31, 1.000000000000000000 ) ) ;
#1283=FACE_OUTER_BOUND ( 'NONE', #4595, .T. ) ;
#1284=EDGE_CURVE ( 'NONE', #921, #4034, #2951, .T. ) ;
#1286=EDGE_LOOP ( 'NONE', ( #2520, #4786, #1113, #206 ) ) ;
#1287=EDGE_LOOP ( 'NONE', ( #51, #5185, #215, #4387 ) ) ;
#1291=CARTESIAN_POINT ( 'NONE',  ( -98.02857808274411866, 84.45434506795672291, -12.00000000000001066 ) ) ;
#1293=DIRECTION ( 'NONE',  ( -5.551115123125772841E-17, 1.848892746611743135E-31, 1.000000000000000000 ) ) ;
#1297=DIRECTION ( 'NONE',  ( -0.4205749795070160557, 0.9072577839912276954, 5.551115123125780853E-17 ) ) ;
#1298=FACE_OUTER_BOUND ( 'NONE', #259, .T. ) ;
#1300=ADVANCED_FACE ( 'NONE', ( #645 ), #4009, .T. ) ;
#1301=EDGE_CURVE ( 'NONE', #2111, #1369, #1525, .T. ) ;
#1307=DIRECTION ( 'NONE',  ( -1.000000000000000000, 0.000000000000000000, 0.000000000000000000 ) ) ;
#1313=PLANE ( 'NONE',  #5033 ) ;
#1314=ORIENTED_EDGE ( 'NONE', *, *, #4623, .F. ) ;
#1316=DIRECTION ( 'NONE',  ( 5.551115123125772841E-17, -1.848892746611743135E-31, -1.000000000000000000 ) ) ;
#1318=DIRECTION ( 'NONE',  ( 5.551115123125772841E-17, -1.848892746611743135E-31, -1.000000000000000000 ) ) ;
#1327=VERTEX_POINT ( 'NONE', #3187 ) ;
#1329=ORIENTED_EDGE ( 'NONE', *, *, #4393, .T. ) ;
#1331=DIRECTION ( 'NONE',  ( 1.000000000000000000, 0.000000000000000000, 0.000000000000000000 ) ) ;
#1341=MANIFOLD_SOLID_BREP ( 'Boss-Extrude1', #2530 ) ;
#1343=VECTOR ( 'NONE', #112, 1000.000000000000000 ) ;
#1344=AXIS2_PLACEMENT_3D ( 'NONE', #284, #4490, #4897 ) ;
#1345=EDGE_LOOP ( 'NONE', ( #4290, #1184, #128, #5421 ) ) ;
#1346=DIRECTION ( 'NONE',  ( 5.551115123125772841E-17, -1.848892746611743135E-31, -1.000000000000000000 ) ) ;
#1347=DIRECTION ( 'NONE',  ( 1.000000000000000000, 0.000000000000000000, 0.000000000000000000 ) ) ;
#1351=ORIENTED_EDGE ( 'NONE', *, *, #5184, .T. ) ;
#1358=( GEOMETRIC_REPRESENTATION_CONTEXT ( 3 ) GLOBAL_UNCERTAINTY_ASSIGNED_CONTEXT ( ( #3647 ) ) GLOBAL_UNIT_ASSIGNED_CONTEXT ( ( #4930, #4844, #4062 ) ) REPRESENTATION_CONTEXT ( 'NONE', 'WORKASPACE' ) );
#1363=ORIENTED_EDGE ( 'NONE', *, *, #5123, .T. ) ;
#1368=DIRECTION ( 'NONE',  ( 5.551115123125772841E-17, -1.848892746611743135E-31, -1.000000000000000000 ) ) ;
#1369=VERTEX_POINT ( 'NONE', #4902 ) ;
#1371=LINE ( 'NONE', #3133, #2698 ) ;
#1377=EDGE_CURVE ( 'NONE', #921, #964, #1571, .T. ) ;
#1379=DIRECTION ( 'NONE',  ( 1.000000000000000000, -3.759415251443877817E-31, 5.551115123125772841E-17 ) ) ;
#1385=DIRECTION ( 'NONE',  ( -1.000000000000000000, 0.000000000000000000, 0.000000000000000000 ) ) ;
#1387=DIRECTION ( 'NONE',  ( 5.551115123125772841E-17, -1.848892746611743135E-31, -1.000000000000000000 ) ) ;
#1391=ORIENTED_EDGE ( 'NONE', *, *, #3564, .T. ) ;
#1392=EDGE_CURVE ( 'NONE', #2971, #800, #4592, .T. ) ;
#1393=CIRCLE ( 'NONE', #2352, 14.00000000000002665 ) ;
#1396=CARTESIAN_POINT ( 'NONE',  ( 133.9714219172562366, 80.45434506795683660, -12.00000000000001066 ) ) ;
#1397=DIRECTION ( 'NONE',  ( 5.551115123125772841E-17, -1.848892746611743135E-31, -1.000000000000000000 ) ) ;
#1408=ORIENTED_EDGE ( 'NONE', *, *, #3721, .T. ) ;
#1416=LINE ( 'NONE', #3218, #4854 ) ;
#1420=CARTESIAN_POINT ( 'NONE',  ( 139.2214219172562366, 80.45434506795679397, -26.84924240491753977 ) ) ;
#1426=AXIS2_PLACEMENT_3D ( 'NONE', #1916, #5210, #1945 ) ;
#1428=ORIENTED_EDGE ( 'NONE', *, *, #2582, .F. ) ;
#1436=EDGE_CURVE ( 'NONE', #4871, #3515, #5410, .T. ) ;
#1437=AXIS2_PLACEMENT_3D ( 'NONE', #4217, #1023, #4327 ) ;
#1439=EDGE_CURVE ( 'NONE', #664, #3905, #3406, .T. ) ;
#1440=AXIS2_PLACEMENT_3D ( 'NONE', #5013, #4184, #5044 ) ;
#1453=DIRECTION ( 'NONE',  ( -1.000000000000000000, 0.000000000000000000, -7.228014483236656373E-17 ) ) ;
#1455=CARTESIAN_POINT ( 'NONE',  ( 133.9714219172562366, -21.54565493204319182, -2.000000000000001776 ) ) ;
#1459=ORIENTED_EDGE ( 'NONE', *, *, #1534, .T. ) ;
#1462=CARTESIAN_POINT ( 'NONE',  ( 151.9714219172563219, 84.45434506795673713, 152.0000000000001990 ) ) ;
#1467=CARTESIAN_POINT ( 'NONE',  ( 151.9714219172562935, -25.54565493204309234, -5.551115123125782702E-14 ) ) ;
#1469=DIRECTION ( 'NONE',  ( -1.000000000000000000, 0.000000000000000000, 0.000000000000000000 ) ) ;
#1474=DIRECTION ( 'NONE',  ( -1.000000000000000000, 0.000000000000000000, -7.228014483236656373E-17 ) ) ;
#1476=DIRECTION ( 'NONE',  ( 5.551115123125772841E-17, -1.848892746611743135E-31, -1.000000000000000000 ) ) ;
#1477=PLANE ( 'NONE',  #2573 ) ;
#1485=DIRECTION ( 'NONE',  ( -1.000000000000000000, 0.000000000000000000, -5.551115123125782702E-17 ) ) ;
#1486=VERTEX_POINT ( 'NONE', #2835 ) ;
#1489=LINE ( 'NONE', #200, #2003 ) ;
#1490=DIRECTION ( 'NONE',  ( -0.4205749795070160002, 0.9072577839912275843, 5.551115123125780237E-17 ) ) ;
#1491=CARTESIAN_POINT ( 'NONE',  ( 133.9714219172562650, 80.45434506795683660, -2.000000000000001776 ) ) ;
#1492=DIRECTION ( 'NONE',  ( -5.551115123125772841E-17, 1.848892746611743135E-31, 1.000000000000000000 ) ) ;
#1493=VERTEX_POINT ( 'NONE', #2509 ) ;
#1494=LINE ( 'NONE', #4149, #372 ) ;
#1497=DIRECTION ( 'NONE',  ( 5.551115123125772841E-17, -1.848892746611743354E-31, -1.000000000000000000 ) ) ;
#1498=EDGE_CURVE ( 'NONE', #2521, #3281, #466, .T. ) ;
#1505=ORIENTED_EDGE ( 'NONE', *, *, #1663, .F. ) ;
#1508=AXIS2_PLACEMENT_3D ( 'NONE', #4653, #4245, #4981 ) ;
#1509=DIRECTION ( 'NONE',  ( -5.551115123125772841E-17, 1.848892746611743135E-31, 1.000000000000000000 ) ) ;
#1515=AXIS2_PLACEMENT_3D ( 'NONE', #3770, #4, #4625 ) ;
#1517=DIRECTION ( 'NONE',  ( 0.4205749795070158337, 0.9072577839912276954, 0.000000000000000000 ) ) ;
#1523=CARTESIAN_POINT ( 'NONE',  ( 133.9714219172562366, 80.45434506795679397, -26.84924240491753977 ) ) ;
#1525=LINE ( 'NONE', #2793, #4101 ) ;
#1526=DIRECTION ( 'NONE',  ( -5.551115123125772841E-17, 1.848892746611743135E-31, 1.000000000000000000 ) ) ;
#1531=DIRECTION ( 'NONE',  ( -1.000000000000000000, 0.000000000000000000, 0.000000000000000000 ) ) ;
#1534=EDGE_CURVE ( 'NONE', #483, #3766, #4570, .T. ) ;
#1539=DIRECTION ( 'NONE',  ( 1.000000000000000000, 0.000000000000000000, 5.551115123125782702E-17 ) ) ;
#1543=ORIENTED_EDGE ( 'NONE', *, *, #3666, .F. ) ;
#1545=ORIENTED_EDGE ( 'NONE', *, *, #5330, .F. ) ;
#1548=EDGE_LOOP ( 'NONE', ( #627, #510, #4173 ) ) ;
#1550=ORIENTED_EDGE ( 'NONE', *, *, #2774, .T. ) ;
#1551=CARTESIAN_POINT ( 'NONE',  ( -84.02857808274400497, -39.54565493204319893, -11.99999999999984368 ) ) ;
#1553=DIRECTION ( 'NONE',  ( 1.000000000000000000, 0.000000000000000000, 5.551115123125777155E-17 ) ) ;
#1554=CARTESIAN_POINT ( 'NONE',  ( -84.02857808274407603, 84.45434506795682239, -11.99999999999995559 ) ) ;
#1555=DIRECTION ( 'NONE',  ( -2.523234146875361914E-16, -1.000000000000000000, -1.456973175402238023E-31 ) ) ;
#1558=DIRECTION ( 'NONE',  ( -5.551115123125772841E-17, 1.848892746611743135E-31, 1.000000000000000000 ) ) ;
#1561=AXIS2_PLACEMENT_3D ( 'NONE', #3367, #2976, #4600 ) ;
#1562=AXIS2_PLACEMENT_3D ( 'NONE', #1455, #5135, #2693 ) ;
#1567=ORIENTED_EDGE ( 'NONE', *, *, #567, .F. ) ;
#1569=VERTEX_POINT ( 'NONE', #2619 ) ;
#1571=LINE ( 'NONE', #3642, #3907 ) ;
#1572=CARTESIAN_POINT ( 'NONE',  ( -80.02857808274410445, -21.54565493204321669, -9.999999999999953815 ) ) ;
#1576=DIRECTION ( 'NONE',  ( -1.000000000000000000, 0.000000000000000000, -8.260587980841909197E-17 ) ) ;
#1577=CARTESIAN_POINT ( 'NONE',  ( -98.02857808274411866, -25.54565493204307813, -11.99999999999995559 ) ) ;
#1581=CARTESIAN_POINT ( 'NONE',  ( 133.9714219172562366, 80.45434506795679397, -26.84924240491753977 ) ) ;
#1584=CARTESIAN_POINT ( 'NONE',  ( -84.02857808274413287, 84.45434506795682239, -5.551115123125782702E-14 ) ) ;
#1598=ORIENTED_EDGE ( 'NONE', *, *, #1060, .T. ) ;
#1602=FACE_OUTER_BOUND ( 'NONE', #1128, .T. ) ;
#1603=CARTESIAN_POINT ( 'NONE',  ( -98.02857808274411866, -25.54565493204307813, -11.99999999999995559 ) ) ;
#1604=EDGE_CURVE ( 'NONE', #3069, #5397, #106, .T. ) ;
#1606=CARTESIAN_POINT ( 'NONE',  ( 133.9714219172562650, 80.45434506795683660, -2.000000000000001776 ) ) ;
#1607=VERTEX_POINT ( 'NONE', #23 ) ;
#1608=ORIENTED_EDGE ( 'NONE', *, *, #3563, .F. ) ;
#1611=DIRECTION ( 'NONE',  ( -0.4205749795070160557, 0.9072577839912276954, 5.551115123125780853E-17 ) ) ;
#1612=AXIS2_PLACEMENT_3D ( 'NONE', #3970, #2266, #1771 ) ;
#1616=VECTOR ( 'NONE', #912, 1000.000000000000000 ) ;
#1617=CARTESIAN_POINT ( 'NONE',  ( 133.9714219172562366, -21.54565493204319182, -26.84924240491753977 ) ) ;
#1620=VECTOR ( 'NONE', #3761, 1000.000000000000000 ) ;
#1625=CARTESIAN_POINT ( 'NONE',  ( 135.7157751673381085, -16.59391465826787027, -9.999999999999953815 ) ) ;
#1626=CYLINDRICAL_SURFACE ( 'NONE', #2411, 14.00000000000002665 ) ;
#1629=FACE_OUTER_BOUND ( 'NONE', #406, .T. ) ;
#1631=DIRECTION ( 'NONE',  ( 5.551115123125772841E-17, -1.848892746611743135E-31, -1.000000000000000000 ) ) ;
#1633=EDGE_LOOP ( 'NONE', ( #2754, #1391, #4723 ) ) ;
#1637=LINE ( 'NONE', #1743, #213 ) ;
#1644=CARTESIAN_POINT ( 'NONE',  ( -77.37696704867106234, 84.98551036222526989, -9.999999999999953815 ) ) ;
#1649=CARTESIAN_POINT ( 'NONE',  ( 132.2270686671743931, -26.49739520581860575, -11.99999999999990052 ) ) ;
#1650=CARTESIAN_POINT ( 'NONE',  ( -84.02857808274407603, 84.45434506795682239, -11.99999999999995559 ) ) ;
#1651=DIRECTION ( 'NONE',  ( 5.551115123125772841E-17, -1.848892746611743135E-31, -1.000000000000000000 ) ) ;
#1655=ORIENTED_EDGE ( 'NONE', *, *, #1834, .F. ) ;
#1659=FACE_OUTER_BOUND ( 'NONE', #1345, .T. ) ;
#1663=EDGE_CURVE ( 'NONE', #4330, #1984, #5101, .T. ) ;
#1664=EDGE_CURVE ( 'NONE', #4404, #1665, #1393, .T. ) ;
#1665=VERTEX_POINT ( 'NONE', #2147 ) ;
#1668=ORIENTED_EDGE ( 'NONE', *, *, #993, .T. ) ;
#1669=DIRECTION ( 'NONE',  ( -1.261617073437686134E-16, 1.000000000000000000, 1.232595164407830946E-31 ) ) ;
#1672=CARTESIAN_POINT ( 'NONE',  ( -84.02857808274403340, 98.45434506795682239, -5.551115123125782702E-14 ) ) ;
#1674=EDGE_CURVE ( 'NONE', #3692, #486, #5136, .T. ) ;
#1675=EDGE_LOOP ( 'NONE', ( #315, #4754, #4352, #5255 ) ) ;
#1676=VERTEX_POINT ( 'NONE', #3874 ) ;
#1677=VECTOR ( 'NONE', #1387, 1000.000000000000000 ) ;
#1678=VERTEX_POINT ( 'NONE', #1260 ) ;
#1684=VECTOR ( 'NONE', #4117, 1000.000000000000000 ) ;
#1687=DIRECTION ( 'NONE',  ( 0.9072577839912275843, 0.4205749795070160002, 1.110223024625155801E-16 ) ) ;
#1690=VECTOR ( 'NONE', #3423, 1000.000000000000000 ) ;
#1691=EDGE_LOOP ( 'NONE', ( #4106, #1608, #1655, #2367 ) ) ;
#1693=ORIENTED_EDGE ( 'NONE', *, *, #3729, .F. ) ;
#1699=VECTOR ( 'NONE', #1297, 999.9999999999998863 ) ;
#1702=VECTOR ( 'NONE', #1611, 999.9999999999998863 ) ;
#1704=PRODUCT ( 'Stainless Steel Outer Shield Cover', 'Stainless Steel Outer Shield Cover', '', ( #5183 ) ) ;
#1705=LINE ( 'NONE', #2094, #3463 ) ;
#1708=CARTESIAN_POINT ( 'NONE',  ( 131.3198108831832656, 84.98551036222518462, -10.00000000000000888 ) ) ;
#1713=CARTESIAN_POINT ( 'NONE',  ( -80.02857808274401918, 80.45434506795689344, -12.00000000000001066 ) ) ;
#1718=CARTESIAN_POINT ( 'NONE',  ( -74.77857808274418971, -21.54565493204320248, -2.000000000000001332 ) ) ;
#1723=ORIENTED_EDGE ( 'NONE', *, *, #720, .T. ) ;
#1726=AXIS2_PLACEMENT_3D ( 'NONE', #593, #1013, #1474 ) ;
#1736=EDGE_CURVE ( 'NONE', #1160, #4218, #729, .T. ) ;
#1739=ORIENTED_EDGE ( 'NONE', *, *, #2854, .F. ) ;
#1740=ORIENTED_EDGE ( 'NONE', *, *, #2176, .T. ) ;
#1741=DIRECTION ( 'NONE',  ( 5.551115123125772841E-17, -1.848892746611743354E-31, -1.000000000000000000 ) ) ;
#1743=CARTESIAN_POINT ( 'NONE',  ( -74.02857808274416129, -21.54565493204321669, -2.000000000000001332 ) ) ;
#1744=DIRECTION ( 'NONE',  ( 1.261617073437686134E-16, -1.000000000000000000, -1.232595164407830946E-31 ) ) ;
#1758=DIRECTION ( 'NONE',  ( 0.4205749795070160557, -0.9072577839912276954, -5.551115123125780853E-17 ) ) ;
#1766=ORIENTED_EDGE ( 'NONE', *, *, #1870, .T. ) ;
#1770=DIRECTION ( 'NONE',  ( -0.4205749795070160557, 0.9072577839912276954, 5.551115123125780853E-17 ) ) ;
#1771=DIRECTION ( 'NONE',  ( -1.000000000000000000, 0.000000000000000000, 0.000000000000000000 ) ) ;
#1773=CARTESIAN_POINT ( 'NONE',  ( 133.9714219172562650, 80.45434506795683660, -2.000000000000001776 ) ) ;
#1776=EDGE_CURVE ( 'NONE', #4528, #3229, #1494, .T. ) ;
#1777=CARTESIAN_POINT ( 'NONE',  ( 151.9714219172563219, 84.45434506795677976, -5.551115123125782702E-14 ) ) ;
#1780=ORIENTED_EDGE ( 'NONE', *, *, #3960, .T. ) ;
#1781=VECTOR ( 'NONE', #2974, 1000.000000000000000 ) ;
#1784=CARTESIAN_POINT ( 'NONE',  ( -78.28422483266226095, 85.40608534173227895, -10.00000000000006395 ) ) ;
#1785=AXIS2_PLACEMENT_3D ( 'NONE', #1491, #2815, #2846 ) ;
#1786=( GEOMETRIC_REPRESENTATION_CONTEXT ( 3 ) GLOBAL_UNCERTAINTY_ASSIGNED_CONTEXT ( ( #3590 ) ) GLOBAL_UNIT_ASSIGNED_CONTEXT ( ( #5203, #2686, #5280 ) ) REPRESENTATION_CONTEXT ( 'NONE', 'WORKASPACE' ) );
#1795=CARTESIAN_POINT ( 'NONE',  ( 151.9714219172562935, 84.45434506795673713, -11.99999999999995559 ) ) ;
#1797=VECTOR ( 'NONE', #211, 1000.000000000000000 ) ;
#1798=AXIS2_PLACEMENT_3D ( 'NONE', #3324, #1277, #41 ) ;
#1799=VERTEX_POINT ( 'NONE', #4847 ) ;
#1800=ORIENTED_EDGE ( 'NONE', *, *, #5103, .T. ) ;
#1808=DIRECTION ( 'NONE',  ( 5.551115123125772841E-17, -1.848892746611743135E-31, -1.000000000000000000 ) ) ;
#1810=FACE_OUTER_BOUND ( 'NONE', #2145, .T. ) ;
#1816=ORIENTED_EDGE ( 'NONE', *, *, #2103, .F. ) ;
#1834=EDGE_CURVE ( 'NONE', #1160, #2642, #4755, .T. ) ;
#1838=EDGE_CURVE ( 'NONE', #3404, #783, #3435, .T. ) ;
#1839=EDGE_CURVE ( 'NONE', #4953, #1676, #2123, .T. ) ;
#1840=ORIENTED_EDGE ( 'NONE', *, *, #1838, .T. ) ;
#1849=CARTESIAN_POINT ( 'NONE',  ( 131.3198108831832656, 84.98551036222518462, -10.00000000000000888 ) ) ;
#1855=DIRECTION ( 'NONE',  ( 5.551115123125772841E-17, -1.848892746611743135E-31, -1.000000000000000000 ) ) ;
#1857=DIRECTION ( 'NONE',  ( 1.000000000000000000, 0.000000000000000000, 0.000000000000000000 ) ) ;
#1860=VECTOR ( 'NONE', #1558, 1000.000000000000000 ) ;
#1864=ADVANCED_FACE ( 'NONE', ( #2079 ), #4253, .T. ) ;
#1866=AXIS2_PLACEMENT_3D ( 'NONE', #2020, #4139, #4167 ) ;
#1869=ORIENTED_EDGE ( 'NONE', *, *, #2944, .F. ) ;
#1870=EDGE_CURVE ( 'NONE', #3390, #4488, #3186, .T. ) ;
#1873=AXIS2_PLACEMENT_3D ( 'NONE', #3403, #804, #887 ) ;
#1877=CIRCLE ( 'NONE', #1262, 6.000000000000032863 ) ;
#1878=ORIENTED_EDGE ( 'NONE', *, *, #3507, .F. ) ;
#1881=CARTESIAN_POINT ( 'NONE',  ( -82.68018911681710392, 75.92317977368848858, -9.999999999999953815 ) ) ;
#1882=FACE_OUTER_BOUND ( 'NONE', #109, .T. ) ;
#1883=CIRCLE ( 'NONE', #3815, 5.250000000000004441 ) ;
#1885=CARTESIAN_POINT ( 'NONE',  ( 137.9714219172562366, 84.45434506795687923, -12.00000000000001066 ) ) ;
#1887=VECTOR ( 'NONE', #2790, 1000.000000000000000 ) ;
#1891=PLANE ( 'NONE',  #2761 ) ;
#1892=CARTESIAN_POINT ( 'NONE',  ( 137.9714219172561513, 98.45434506795687923, -12.00000000000006573 ) ) ;
#1899=EDGE_LOOP ( 'NONE', ( #3785, #3231, #671, #1543, #3257, #2235, #2137, #1668 ) ) ;
#1900=CARTESIAN_POINT ( 'NONE',  ( -80.02857808274410445, -21.54565493204320248, -26.84924240491759662 ) ) ;
#1905=FACE_BOUND ( 'NONE', #4578, .T. ) ;
#1907=DIRECTION ( 'NONE',  ( 5.551115123125772841E-17, -1.848892746611743135E-31, -1.000000000000000000 ) ) ;
#1908=CARTESIAN_POINT ( 'NONE',  ( -98.02857808274411866, 84.45434506795672291, 5.551115123125782702E-14 ) ) ;
#1910=LINE ( 'NONE', #177, #204 ) ;
#1916=CARTESIAN_POINT ( 'NONE',  ( -78.28422483266226095, 85.40608534173227895, -10.00000000000006395 ) ) ;
#1925=ORIENTED_EDGE ( 'NONE', *, *, #1036, .T. ) ;
#1926=CARTESIAN_POINT ( 'NONE',  ( 137.9714219172561798, -39.54565493204318471, -5.551115123125782702E-14 ) ) ;
#1930=VERTEX_POINT ( 'NONE', #3351 ) ;
#1933=CARTESIAN_POINT ( 'NONE',  ( -84.02857808274400497, -39.54565493204319893, -11.99999999999984368 ) ) ;
#1934=CARTESIAN_POINT ( 'NONE',  ( 131.3198108831831519, -26.07682022631159668, -12.00000000000001066 ) ) ;
#1935=EDGE_CURVE ( 'NONE', #3692, #2650, #455, .T. ) ;
#1938=ADVANCED_FACE ( 'NONE', ( #3326 ), #4688, .T. ) ;
#1941=DIRECTION ( 'NONE',  ( -5.551115123125772841E-17, 1.848892746611743135E-31, 1.000000000000000000 ) ) ;
#1945=DIRECTION ( 'NONE',  ( -0.4205749795070158337, -0.9072577839912276954, 0.000000000000000000 ) ) ;
#1947=CARTESIAN_POINT ( 'NONE',  ( 151.9714219172563219, 84.45434506795677976, -5.551115123125782702E-14 ) ) ;
#1950=DIRECTION ( 'NONE',  ( 0.4205749795070158337, 0.9072577839912276954, 0.000000000000000000 ) ) ;
#1954=ORIENTED_EDGE ( 'NONE', *, *, #2417, .F. ) ;
#1961=ORIENTED_EDGE ( 'NONE', *, *, #2485, .F. ) ;
#1962=VECTOR ( 'NONE', #4882, 999.9999999999998863 ) ;
#1968=DIRECTION ( 'NONE',  ( 1.000000000000000000, 0.000000000000000000, 0.000000000000000000 ) ) ;
#1972=EDGE_CURVE ( 'NONE', #4236, #4708, #4929, .T. ) ;
#1973=FACE_OUTER_BOUND ( 'NONE', #1286, .T. ) ;
#1977=VECTOR ( 'NONE', #10, 999.9999999999998863 ) ;
#1979=VECTOR ( 'NONE', #5235, 1000.000000000000000 ) ;
#1980=CARTESIAN_POINT ( 'NONE',  ( 131.3198108831832087, -26.07682022631159668, -10.00000000000000888 ) ) ;
#1983=LINE ( 'NONE', #2801, #3462 ) ;
#1984=VERTEX_POINT ( 'NONE', #3891 ) ;
#1989=ORIENTED_EDGE ( 'NONE', *, *, #3060, .T. ) ;
#1994=DIRECTION ( 'NONE',  ( 0.9072577839912275843, 0.4205749795070160002, 1.110223024625155801E-16 ) ) ;
#1996=LINE ( 'NONE', #3396, #3113 ) ;
#1997=EDGE_LOOP ( 'NONE', ( #4025, #2747, #1259, #4606 ) ) ;
#2003=VECTOR ( 'NONE', #3266, 1000.000000000000000 ) ;
#2011=ORIENTED_EDGE ( 'NONE', *, *, #2435, .F. ) ;
#2015=EDGE_CURVE ( 'NONE', #3533, #496, #122, .T. ) ;
#2018=ORIENTED_EDGE ( 'NONE', *, *, #5259, .F. ) ;
#2020=CARTESIAN_POINT ( 'NONE',  ( 133.9714219172562366, -21.54565493204319182, -12.00000000000006573 ) ) ;
#2021=DIRECTION ( 'NONE',  ( -1.000000000000000000, 3.759415251443877379E-31, -5.551115123125772841E-17 ) ) ;
#2027=LINE ( 'NONE', #3682, #821 ) ;
#2037=ORIENTED_EDGE ( 'NONE', *, *, #499, .F. ) ;
#2040=AXIS2_PLACEMENT_3D ( 'NONE', #451, #3378, #892 ) ;
#2045=DIRECTION ( 'NONE',  ( 5.551115123125772841E-17, -1.848892746611743135E-31, -1.000000000000000000 ) ) ;
#2048=VECTOR ( 'NONE', #4447, 1000.000000000000000 ) ;
#2050=ORIENTED_EDGE ( 'NONE', *, *, #2176, .F. ) ;
#2055=CARTESIAN_POINT ( 'NONE',  ( -80.02857808274418971, -21.54565493204321669, -2.000000000000001776 ) ) ;
#2056=CIRCLE ( 'NONE', #3380, 14.00000000000002665 ) ;
#2057=VECTOR ( 'NONE', #1293, 1000.000000000000000 ) ;
#2058=CIRCLE ( 'NONE', #126, 14.00000000000002665 ) ;
#2065=EDGE_LOOP ( 'NONE', ( #4076, #3044, #2483, #1693, #2979, #3093, #1816, #2995 ) ) ;
#2068=ORIENTED_EDGE ( 'NONE', *, *, #3416, .F. ) ;
#2073=DIRECTION ( 'NONE',  ( -0.9072577839912275843, -0.4205749795070160002, -1.110223024625155801E-16 ) ) ;
#2074=ORIENTED_EDGE ( 'NONE', *, *, #1839, .T. ) ;
#2078=EDGE_CURVE ( 'NONE', #3069, #3692, #4743, .T. ) ;
#2079=FACE_OUTER_BOUND ( 'NONE', #2065, .T. ) ;
#2085=DIRECTION ( 'NONE',  ( -5.551115123125772841E-17, 1.848892746611743135E-31, 1.000000000000000000 ) ) ;
#2088=VECTOR ( 'NONE', #2203, 1000.000000000000114 ) ;
#2091=CARTESIAN_POINT ( 'NONE',  ( 133.9714219172562366, -21.54565493204323090, -9.999999999999841904 ) ) ;
#2093=EDGE_LOOP ( 'NONE', ( #2281, #3488, #4945 ) ) ;
#2094=CARTESIAN_POINT ( 'NONE',  ( 131.3198108831831519, -26.07682022631159668, -12.00000000000001066 ) ) ;
#2103=EDGE_CURVE ( 'NONE', #5397, #4871, #3453, .T. ) ;
#2105=EDGE_CURVE ( 'NONE', #850, #3157, #3152, .T. ) ;
#2111=VERTEX_POINT ( 'NONE', #5251 ) ;
#2112=ORIENTED_EDGE ( 'NONE', *, *, #1834, .T. ) ;
#2114=SHAPE_REPRESENTATION_RELATIONSHIP ( 'NONE' , 'NONE' ,  #3079, #4432 ) ;
#2117=DIRECTION ( 'NONE',  ( 5.551115123125772841E-17, -1.848892746611743135E-31, -1.000000000000000000 ) ) ;
#2122=CARTESIAN_POINT ( 'NONE',  ( -74.02857808274417550, -21.54565493204321669, -2.000000000000001332 ) ) ;
#2123=CIRCLE ( 'NONE', #711, 6.000000000000032863 ) ;
#2125=ORIENTED_EDGE ( 'NONE', *, *, #1436, .T. ) ;
#2130=DIRECTION ( 'NONE',  ( 5.551115123125772841E-17, -1.848892746611743135E-31, -1.000000000000000000 ) ) ;
#2133=VECTOR ( 'NONE', #1517, 1000.000000000000114 ) ;
#2134=ADVANCED_FACE ( 'NONE', ( #1602 ), #4523, .F. ) ;
#2135=CARTESIAN_POINT ( 'NONE',  ( -98.02857808274411866, 84.45434506795672291, 5.551115123125782702E-14 ) ) ;
#2137=ORIENTED_EDGE ( 'NONE', *, *, #3687, .T. ) ;
#2138=AXIS2_PLACEMENT_3D ( 'NONE', #1554, #5252, #4469 ) ;
#2142=CARTESIAN_POINT ( 'NONE',  ( 137.9714219172560945, -39.54565493204318471, -11.99999999999995559 ) ) ;
#2144=AXIS2_PLACEMENT_3D ( 'NONE', #3765, #1687, #412 ) ;
#2145=EDGE_LOOP ( 'NONE', ( #4835, #1840, #1800, #5117 ) ) ;
#2147=CARTESIAN_POINT ( 'NONE',  ( -84.02857808274403340, 98.45434506795682239, -5.551115123125782702E-14 ) ) ;
#2149=VECTOR ( 'NONE', #2547, 1000.000000000000000 ) ;
#2153=AXIS2_PLACEMENT_3D ( 'NONE', #1708, #2073, #1222 ) ;
#2158=CARTESIAN_POINT ( 'NONE',  ( 128.7214219172562366, -21.54565493204319182, -12.00000000000006573 ) ) ;
#2161=ORIENTED_EDGE ( 'NONE', *, *, #795, .T. ) ;
#2167=DIRECTION ( 'NONE',  ( 1.000000000000000000, -3.759415251443877379E-31, 5.551115123125772841E-17 ) ) ;
#2168=ORIENTED_EDGE ( 'NONE', *, *, #2512, .F. ) ;
#2176=EDGE_CURVE ( 'NONE', #5368, #483, #4412, .T. ) ;
#2178=ORIENTED_EDGE ( 'NONE', *, *, #1498, .F. ) ;
#2182=EDGE_CURVE ( 'NONE', #496, #2670, #4005, .T. ) ;
#2186=DIRECTION ( 'NONE',  ( 5.551115123125772841E-17, -1.848892746611743135E-31, -1.000000000000000000 ) ) ;
#2188=ADVANCED_FACE ( 'NONE', ( #2348 ), #287, .F. ) ;
#2190=ORIENTED_EDGE ( 'NONE', *, *, #4064, .F. ) ;
#2194=CARTESIAN_POINT ( 'NONE',  ( 127.9714219172561940, -21.54565493204319182, -2.000000000000002220 ) ) ;
#2196=CARTESIAN_POINT ( 'NONE',  ( -98.02857808274411866, 84.45434506795672291, 152.0000000000001990 ) ) ;
#2201=ORIENTED_EDGE ( 'NONE', *, *, #3959, .T. ) ;
#2202=EDGE_LOOP ( 'NONE', ( #4249, #118 ) ) ;
#2203=DIRECTION ( 'NONE',  ( 0.4205749795070158337, 0.9072577839912276954, 0.000000000000000000 ) ) ;
#2205=ORIENTED_EDGE ( 'NONE', *, *, #4780, .F. ) ;
#2213=ORIENTED_EDGE ( 'NONE', *, *, #5430, .F. ) ;
#2216=VECTOR ( 'NONE', #2607, 1000.000000000000000 ) ;
#2218=DIRECTION ( 'NONE',  ( -1.000000000000000000, 0.000000000000000000, 0.000000000000000000 ) ) ;
#2219=LINE ( 'NONE', #2194, #4166 ) ;
#2228=VERTEX_POINT ( 'NONE', #1577 ) ;
#2230=SHAPE_DEFINITION_REPRESENTATION ( #311, #3079 ) ;
#2231=VECTOR ( 'NONE', #254, 1000.000000000000000 ) ;
#2235=ORIENTED_EDGE ( 'NONE', *, *, #2813, .F. ) ;
#2241=AXIS2_PLACEMENT_3D ( 'NONE', #956, #1476, #4822 ) ;
#2243=ORIENTED_EDGE ( 'NONE', *, *, #4924, .T. ) ;
#2247=CARTESIAN_POINT ( 'NONE',  ( -84.02857808274407603, 84.45434506795682239, -11.99999999999995559 ) ) ;
#2249=ORIENTED_EDGE ( 'NONE', *, *, #1211, .F. ) ;
#2251=EDGE_CURVE ( 'NONE', #1066, #3281, #5365, .T. ) ;
#2257=EDGE_LOOP ( 'NONE', ( #3465, #808, #1925, #2697 ) ) ;
#2258=DIRECTION ( 'NONE',  ( 5.551115123125772841E-17, -1.848892746611743135E-31, -1.000000000000000000 ) ) ;
#2259=DIRECTION ( 'NONE',  ( 0.4205749795070160557, -0.9072577839912276954, -5.551115123125780853E-17 ) ) ;
#2264=CARTESIAN_POINT ( 'NONE',  ( -84.02857808274407603, 84.45434506795682239, -11.99999999999995559 ) ) ;
#2266=DIRECTION ( 'NONE',  ( 5.551115123125772841E-17, -1.848892746611743135E-31, -1.000000000000000000 ) ) ;
#2267=FACE_OUTER_BOUND ( 'NONE', #4746, .T. ) ;
#2270=CARTESIAN_POINT ( 'NONE',  ( -84.02857808274397655, -39.54565493204319893, 152.0000000000000853 ) ) ;
#2275=DIRECTION ( 'NONE',  ( 3.204747427460360459E-31, -1.000000000000000000, 1.848892746611743354E-31 ) ) ;
#2276=ADVANCED_FACE ( 'NONE', ( #1165 ), #2563, .T. ) ;
#2281=ORIENTED_EDGE ( 'NONE', *, *, #1674, .F. ) ;
#2282=FACE_OUTER_BOUND ( 'NONE', #793, .T. ) ;
#2283=DIRECTION ( 'NONE',  ( -5.551115123125772841E-17, 1.848892746611743135E-31, 1.000000000000000000 ) ) ;
#2284=ORIENTED_EDGE ( 'NONE', *, *, #5398, .T. ) ;
#2285=VERTEX_POINT ( 'NONE', #2158 ) ;
#2287=CARTESIAN_POINT ( 'NONE',  ( -80.02857808274404761, 80.45434506795689344, -9.999999999999841904 ) ) ;
#2288=DIRECTION ( 'NONE',  ( 5.551115123125772841E-17, -1.848892746611743135E-31, -1.000000000000000000 ) ) ;
#2289=FACE_OUTER_BOUND ( 'NONE', #1287, .T. ) ;
#2295=ADVANCED_FACE ( 'NONE', ( #2539 ), #3833, .T. ) ;
#2304=VECTOR ( 'NONE', #2787, 1000.000000000000000 ) ;
#2316=ORIENTED_EDGE ( 'NONE', *, *, #5428, .T. ) ;
#2318=FACE_BOUND ( 'NONE', #4947, .T. ) ;
#2320=CARTESIAN_POINT ( 'NONE',  ( -82.68018911681723182, -17.01448963777485446, -12.00000000000006573 ) ) ;
#2321=AXIS2_PLACEMENT_3D ( 'NONE', #2609, #491, #2167 ) ;
#2326=FACE_OUTER_BOUND ( 'NONE', #1899, .T. ) ;
#2329=DIRECTION ( 'NONE',  ( -1.000000000000000000, 0.000000000000000000, 0.000000000000000000 ) ) ;
#2337=VERTEX_POINT ( 'NONE', #6 ) ;
#2344=EDGE_CURVE ( 'NONE', #964, #577, #4843, .T. ) ;
#2345=ORIENTED_EDGE ( 'NONE', *, *, #3804, .F. ) ;
#2347=DIRECTION ( 'NONE',  ( 5.551115123125772841E-17, -1.848892746611743135E-31, -1.000000000000000000 ) ) ;
#2348=FACE_OUTER_BOUND ( 'NONE', #605, .T. ) ;
#2349=DIRECTION ( 'NONE',  ( -1.261617073437686134E-16, 1.000000000000000000, 1.232595164407830946E-31 ) ) ;
#2350=DIRECTION ( 'NONE',  ( 5.551115123125772841E-17, -1.848892746611743135E-31, -1.000000000000000000 ) ) ;
#2352=AXIS2_PLACEMENT_3D ( 'NONE', #2968, #1346, #468 ) ;
#2354=CYLINDRICAL_SURFACE ( 'NONE', #4517, 14.00000000000002665 ) ;
#2356=DIRECTION ( 'NONE',  ( 5.551115123125772841E-17, -1.848892746611743135E-31, -1.000000000000000000 ) ) ;
#2357=AXIS2_PLACEMENT_3D ( 'NONE', #4937, #1178, #4538 ) ;
#2367=ORIENTED_EDGE ( 'NONE', *, *, #1736, .T. ) ;
#2368=CARTESIAN_POINT ( 'NONE',  ( 137.9714219172562366, -25.54565493204319182, -5.551115123125782702E-14 ) ) ;
#2370=ADVANCED_FACE ( 'NONE', ( #5055 ), #3320, .F. ) ;
#2373=ADVANCED_FACE ( 'NONE', ( #3402, #1298 ), #4141, .F. ) ;
#2376=CARTESIAN_POINT ( 'NONE',  ( -85.27857808274418971, -21.54565493204320248, -2.000000000000002220 ) ) ;
#2382=CARTESIAN_POINT ( 'NONE',  ( 132.2270686671743647, -26.49739520581860219, -9.999999999999953815 ) ) ;
#2384=LINE ( 'NONE', #1248, #1620 ) ;
#2385=PLANE ( 'NONE',  #3638 ) ;
#2390=CARTESIAN_POINT ( 'NONE',  ( -74.02857808274409024, -21.54565493204321669, -12.00000000000001066 ) ) ;
#2398=AXIS2_PLACEMENT_3D ( 'NONE', #2368, #5245, #1485 ) ;
#2401=AXIS2_PLACEMENT_3D ( 'NONE', #5066, #4282, #2549 ) ;
#2403=LINE ( 'NONE', #232, #2304 ) ;
#2408=AXIS2_PLACEMENT_3D ( 'NONE', #1885, #4841, #5231 ) ;
#2410=ORIENTED_EDGE ( 'NONE', *, *, #5046, .F. ) ;
#2411=AXIS2_PLACEMENT_3D ( 'NONE', #2869, #772, #2969 ) ;
#2412=DIRECTION ( 'NONE',  ( -1.000000000000000000, 0.000000000000000000, 0.000000000000000000 ) ) ;
#2417=EDGE_CURVE ( 'NONE', #577, #4350, #2736, .T. ) ;
#2419=EDGE_CURVE ( 'NONE', #1042, #5024, #3628, .T. ) ;
#2422=DIRECTION ( 'NONE',  ( 1.000000000000000000, -3.759415251443877379E-31, 5.551115123125772841E-17 ) ) ;
#2425=VERTEX_POINT ( 'NONE', #2874 ) ;
#2435=EDGE_CURVE ( 'NONE', #4710, #774, #2486, .T. ) ;
#2438=APPLICATION_CONTEXT ( 'automotive_design' ) ;
#2439=CARTESIAN_POINT ( 'NONE',  ( 128.7214219172562366, -21.54565493204319182, -26.84924240491753977 ) ) ;
#2446=CARTESIAN_POINT ( 'NONE',  ( -80.02857808274418971, -21.54565493204321669, -2.000000000000001776 ) ) ;
#2448=ADVANCED_FACE ( 'NONE', ( #4737 ), #4681, .F. ) ;
#2449=DIRECTION ( 'NONE',  ( -0.4205749795070158337, -0.9072577839912276954, 0.000000000000000000 ) ) ;
#2453=ORIENTED_EDGE ( 'NONE', *, *, #5046, .T. ) ;
#2458=EDGE_LOOP ( 'NONE', ( #439, #2617, #1265 ) ) ;
#2462=DIRECTION ( 'NONE',  ( -1.261617073437686134E-16, 1.000000000000000000, 1.232595164407830946E-31 ) ) ;
#2463=DIRECTION ( 'NONE',  ( -1.000000000000000000, 0.000000000000000000, 0.000000000000000000 ) ) ;
#2471=LINE ( 'NONE', #1118, #1702 ) ;
#2476=VERTEX_POINT ( 'NONE', #5167 ) ;
#2478=VECTOR ( 'NONE', #1770, 999.9999999999998863 ) ;
#2480=DIRECTION ( 'NONE',  ( -5.551115123125772841E-17, 1.848892746611743135E-31, 1.000000000000000000 ) ) ;
#2482=EDGE_CURVE ( 'NONE', #5024, #1678, #1097, .T. ) ;
#2483=ORIENTED_EDGE ( 'NONE', *, *, #3804, .T. ) ;
#2484=ORIENTED_EDGE ( 'NONE', *, *, #5162, .F. ) ;
#2485=EDGE_CURVE ( 'NONE', #4236, #3749, #5113, .T. ) ;
#2486=CIRCLE ( 'NONE', #108, 6.000000000000032863 ) ;
#2488=DIRECTION ( 'NONE',  ( 1.000000000000000000, -3.759415251443877379E-31, 5.551115123125772841E-17 ) ) ;
#2490=ORIENTED_EDGE ( 'NONE', *, *, #1377, .F. ) ;
#2491=CIRCLE ( 'NONE', #1866, 5.250000000000004441 ) ;
#2494=CARTESIAN_POINT ( 'NONE',  ( -80.02857808274401918, 80.45434506795689344, -12.00000000000001066 ) ) ;
#2495=CARTESIAN_POINT ( 'NONE',  ( -82.68018911681716077, -17.01448963777485446, -9.999999999999953815 ) ) ;
#2497=AXIS2_PLACEMENT_3D ( 'NONE', #1110, #1140, #4056 ) ;
#2498=DIRECTION ( 'NONE',  ( -1.000000000000000000, 0.000000000000000000, 0.000000000000000000 ) ) ;
#2501=CIRCLE ( 'NONE', #125, 5.250000000000031974 ) ;
#2509=CARTESIAN_POINT ( 'NONE',  ( 127.9714219172562508, -21.54565493204319182, -12.00000000000006573 ) ) ;
#2510=FACE_OUTER_BOUND ( 'NONE', #2956, .T. ) ;
#2512=EDGE_CURVE ( 'NONE', #774, #556, #3486, .T. ) ;
#2513=CARTESIAN_POINT ( 'NONE',  ( -78.28422483266226095, 85.40608534173227895, -10.00000000000006395 ) ) ;
#2519=EDGE_CURVE ( 'NONE', #3766, #4657, #4849, .T. ) ;
#2520=ORIENTED_EDGE ( 'NONE', *, *, #2981, .F. ) ;
#2521=VERTEX_POINT ( 'NONE', #2390 ) ;
#2528=DIRECTION ( 'NONE',  ( 5.551115123125772841E-17, -1.848892746611743135E-31, -1.000000000000000000 ) ) ;
#2530=CLOSED_SHELL ( 'NONE', ( #2276, #4948, #5328, #2848, #2912, #3353, #658, #1134, #235, #3956 ) ) ;
#2531=ORIENTED_EDGE ( 'NONE', *, *, #1439, .T. ) ;
#2535=ORIENTED_EDGE ( 'NONE', *, *, #5158, .T. ) ;
#2537=LINE ( 'NONE', #4651, #990 ) ;
#2539=FACE_OUTER_BOUND ( 'NONE', #1691, .T. ) ;
#2540=EDGE_CURVE ( 'NONE', #4195, #3075, #1983, .T. ) ;
#2541=PLANE ( 'NONE',  #1437 ) ;
#2545=PLANE ( 'NONE',  #308 ) ;
#2547=DIRECTION ( 'NONE',  ( 5.551115123125772841E-17, -1.848892746611743135E-31, -1.000000000000000000 ) ) ;
#2549=DIRECTION ( 'NONE',  ( -1.000000000000000000, 0.000000000000000000, -7.228014483236656373E-17 ) ) ;
#2553=VECTOR ( 'NONE', #2462, 1000.000000000000000 ) ;
#2555=ORIENTED_EDGE ( 'NONE', *, *, #5219, .F. ) ;
#2557=CARTESIAN_POINT ( 'NONE',  ( -80.02857808274413287, 80.45434506795689344, -26.84924240491753977 ) ) ;
#2558=EDGE_LOOP ( 'NONE', ( #5193, #5045, #2249, #1329 ) ) ;
#2563=CYLINDRICAL_SURFACE ( 'NONE', #3457, 14.00000000000002665 ) ;
#2566=ORIENTED_EDGE ( 'NONE', *, *, #4924, .F. ) ;
#2567=ORIENTED_EDGE ( 'NONE', *, *, #5259, .T. ) ;
#2569=ORIENTED_EDGE ( 'NONE', *, *, #5103, .F. ) ;
#2572=DIRECTION ( 'NONE',  ( 5.551115123125772841E-17, -1.848892746611743135E-31, -1.000000000000000000 ) ) ;
#2573=AXIS2_PLACEMENT_3D ( 'NONE', #4392, #1497, #3165 ) ;
#2575=ORIENTED_EDGE ( 'NONE', *, *, #4366, .F. ) ;
#2582=EDGE_CURVE ( 'NONE', #534, #4953, #3854, .T. ) ;
#2585=EDGE_CURVE ( 'NONE', #4718, #4330, #4676, .T. ) ;
#2586=CIRCLE ( 'NONE', #3904, 6.000000000000032863 ) ;
#2588=ORIENTED_EDGE ( 'NONE', *, *, #1439, .F. ) ;
#2595=AXIS2_PLACEMENT_3D ( 'NONE', #4899, #4876, #1968 ) ;
#2596=DIRECTION ( 'NONE',  ( 5.551115123125772841E-17, -1.848892746611743354E-31, -1.000000000000000000 ) ) ;
#2600=LINE ( 'NONE', #1795, #4861 ) ;
#2603=ORIENTED_EDGE ( 'NONE', *, *, #644, .T. ) ;
#2604=ADVANCED_FACE ( 'NONE', ( #3399, #3917 ), #86, .T. ) ;
#2607=DIRECTION ( 'NONE',  ( 5.551115123125772841E-17, -1.848892746611743135E-31, -1.000000000000000000 ) ) ;
#2609=CARTESIAN_POINT ( 'NONE',  ( -80.02857808274410445, -21.54565493204321669, -9.999999999999953815 ) ) ;
#2612=CARTESIAN_POINT ( 'NONE',  ( -80.02857808274410445, -21.54565493204320248, -12.00000000000001066 ) ) ;
#2614=CARTESIAN_POINT ( 'NONE',  ( 135.7157751673380801, 75.50260479418143689, -10.00000000000006395 ) ) ;
#2617=ORIENTED_EDGE ( 'NONE', *, *, #2419, .T. ) ;
#2619=CARTESIAN_POINT ( 'NONE',  ( -74.77857808274400497, 80.45434506795689344, -2.000000000000112355 ) ) ;
#2627=VERTEX_POINT ( 'NONE', #4300 ) ;
#2632=CYLINDRICAL_SURFACE ( 'NONE', #4943, 6.000000000000032863 ) ;
#2642=VERTEX_POINT ( 'NONE', #3792 ) ;
#2646=LINE ( 'NONE', #555, #4690 ) ;
#2649=ORIENTED_EDGE ( 'NONE', *, *, #56, .T. ) ;
#2650=VERTEX_POINT ( 'NONE', #3878 ) ;
#2655=CARTESIAN_POINT ( 'NONE',  ( 151.9714219172562935, -25.54565493204309234, -5.551115123125782702E-14 ) ) ;
#2656=CARTESIAN_POINT ( 'NONE',  ( 137.9714219172562082, 98.45434506795683660, 152.0000000000003126 ) ) ;
#2658=FACE_OUTER_BOUND ( 'NONE', #611, .T. ) ;
#2661=CIRCLE ( 'NONE', #2837, 5.250000000000004441 ) ;
#2666=CIRCLE ( 'NONE', #207, 6.000000000000032863 ) ;
#2667=AXIS2_PLACEMENT_3D ( 'NONE', #1086, #4903, #1116 ) ;
#2670=VERTEX_POINT ( 'NONE', #3831 ) ;
#2673=LINE ( 'NONE', #3587, #21 ) ;
#2677=CIRCLE ( 'NONE', #3910, 5.250000000000004441 ) ;
#2679=EDGE_CURVE ( 'NONE', #2642, #864, #3483, .T. ) ;
#2680=EDGE_LOOP ( 'NONE', ( #2531, #4362, #2867, #3010 ) ) ;
#2682=EDGE_CURVE ( 'NONE', #5397, #486, #4272, .T. ) ;
#2684=DIRECTION ( 'NONE',  ( -1.000000000000000000, 3.759415251443877379E-31, -5.551115123125772841E-17 ) ) ;
#2685=EDGE_CURVE ( 'NONE', #3281, #2521, #4763, .T. ) ;
#2686=( NAMED_UNIT ( * ) PLANE_ANGLE_UNIT ( ) SI_UNIT ( $, .RADIAN. ) );
#2687=VERTEX_POINT ( 'NONE', #3063 ) ;
#2688=DIRECTION ( 'NONE',  ( 1.000000000000000000, -3.759415251443877379E-31, 5.551115123125772841E-17 ) ) ;
#2691=DIRECTION ( 'NONE',  ( 5.551115123125772841E-17, -1.848892746611743135E-31, -1.000000000000000000 ) ) ;
#2693=DIRECTION ( 'NONE',  ( 1.000000000000000000, 0.000000000000000000, 8.260587980841931384E-17 ) ) ;
#2697=ORIENTED_EDGE ( 'NONE', *, *, #1284, .T. ) ;
#2698=VECTOR ( 'NONE', #3053, 1000.000000000000114 ) ;
#2699=DIRECTION ( 'NONE',  ( -5.551115123125772841E-17, 1.848892746611743135E-31, 1.000000000000000000 ) ) ;
#2703=ORIENTED_EDGE ( 'NONE', *, *, #617, .T. ) ;
#2711=DIRECTION ( 'NONE',  ( -5.551115123125772841E-17, 1.848892746611743354E-31, 1.000000000000000000 ) ) ;
#2714=LINE ( 'NONE', #2771, #2048 ) ;
#2723=EDGE_LOOP ( 'NONE', ( #4375, #3418, #5247, #2410, #387, #2213, #3178, #1780 ) ) ;
#2734=DIRECTION ( 'NONE',  ( 5.551115123125772841E-17, -1.848892746611743135E-31, -1.000000000000000000 ) ) ;
#2736=CIRCLE ( 'NONE', #1508, 5.250000000000018652 ) ;
#2743=ADVANCED_FACE ( 'NONE', ( #2282 ), #192, .T. ) ;
#2745=EDGE_LOOP ( 'NONE', ( #5059, #1545, #1224, #417, #1739, #2484, #5354, #1274 ) ) ;
#2747=ORIENTED_EDGE ( 'NONE', *, *, #2182, .F. ) ;
#2749=FACE_OUTER_BOUND ( 'NONE', #552, .T. ) ;
#2751=STYLED_ITEM('',(#5458),#3192);
#2752=PLANE ( 'NONE',  #1257 ) ;
#2754=ORIENTED_EDGE ( 'NONE', *, *, #720, .F. ) ;
#2757=CARTESIAN_POINT ( 'NONE',  ( -84.02857808274400497, -39.54565493204319182, -5.551115123125782702E-14 ) ) ;
#2758=FACE_BOUND ( 'NONE', #3750, .T. ) ;
#2760=FACE_OUTER_BOUND ( 'NONE', #2558, .T. ) ;
#2761=AXIS2_PLACEMENT_3D ( 'NONE', #135, #4727, #3577 ) ;
#2767=DIRECTION ( 'NONE',  ( 1.000000000000000000, -3.759415251443877817E-31, 5.551115123125772841E-17 ) ) ;
#2771=CARTESIAN_POINT ( 'NONE',  ( -84.02857808274397655, -39.54565493204319893, 152.0000000000000853 ) ) ;
#2774=EDGE_CURVE ( 'NONE', #2687, #1665, #3121, .T. ) ;
#2776=DIRECTION ( 'NONE',  ( 1.000000000000000000, 0.000000000000000000, 7.228014483236656373E-17 ) ) ;
#2777=EDGE_CURVE ( 'NONE', #1327, #405, #2673, .T. ) ;
#2778=ORIENTED_EDGE ( 'NONE', *, *, #5123, .F. ) ;
#2780=VERTEX_POINT ( 'NONE', #1926 ) ;
#2787=DIRECTION ( 'NONE',  ( 5.551115123125772841E-17, -1.848892746611743135E-31, -1.000000000000000000 ) ) ;
#2790=DIRECTION ( 'NONE',  ( -5.551115123125772841E-17, 1.848892746611743135E-31, 1.000000000000000000 ) ) ;
#2793=CARTESIAN_POINT ( 'NONE',  ( 136.6230329513292361, -17.01448963777488288, -9.999999999999953815 ) ) ;
#2796=DIRECTION ( 'NONE',  ( -5.551115123125772841E-17, 1.848892746611743354E-31, 1.000000000000000000 ) ) ;
#2797=PLANE ( 'NONE',  #1426 ) ;
#2801=CARTESIAN_POINT ( 'NONE',  ( 137.9714219172561513, 98.45434506795689344, -12.00000000000006573 ) ) ;
#2806=DIRECTION ( 'NONE',  ( -5.551115123125772841E-17, 1.848892746611743135E-31, 1.000000000000000000 ) ) ;
#2807=DIRECTION ( 'NONE',  ( 5.551115123125772841E-17, -1.848892746611743135E-31, -1.000000000000000000 ) ) ;
#2813=EDGE_CURVE ( 'NONE', #4708, #3749, #2661, .T. ) ;
#2815=DIRECTION ( 'NONE',  ( 5.551115123125772841E-17, -1.848892746611743135E-31, -1.000000000000000000 ) ) ;
#2822=FACE_OUTER_BOUND ( 'NONE', #2680, .T. ) ;
#2825=FACE_OUTER_BOUND ( 'NONE', #2723, .T. ) ;
#2830=ORIENTED_EDGE ( 'NONE', *, *, #2105, .T. ) ;
#2832=ORIENTED_EDGE ( 'NONE', *, *, #1083, .T. ) ;
#2834=ADVANCED_FACE ( 'NONE', ( #3964 ), #4456, .T. ) ;
#2835=CARTESIAN_POINT ( 'NONE',  ( 131.3198108831832087, -26.07682022631159668, -10.00000000000000888 ) ) ;
#2837=AXIS2_PLACEMENT_3D ( 'NONE', #4353, #2258, #580 ) ;
#2838=CIRCLE ( 'NONE', #3368, 5.250000000000018652 ) ;
#2840=AXIS2_PLACEMENT_3D ( 'NONE', #66, #1631, #3347 ) ;
#2841=CIRCLE ( 'NONE', #641, 5.250000000000018652 ) ;
#2846=DIRECTION ( 'NONE',  ( -1.000000000000000000, 0.000000000000000000, -8.260587980841931384E-17 ) ) ;
#2847=VECTOR ( 'NONE', #2807, 1000.000000000000000 ) ;
#2848=ADVANCED_FACE ( 'NONE', ( #2749 ), #686, .F. ) ;
#2849=AXIS2_PLACEMENT_3D ( 'NONE', #4233, #3819, #495 ) ;
#2850=CARTESIAN_POINT ( 'NONE',  ( 139.2214219172562650, -21.54565493204319182, -26.84924240491753977 ) ) ;
#2853=CARTESIAN_POINT ( 'NONE',  ( 137.9714219172561513, 98.45434506795687923, -12.00000000000006573 ) ) ;
#2854=EDGE_CURVE ( 'NONE', #4218, #2780, #812, .T. ) ;
#2855=AXIS2_PLACEMENT_3D ( 'NONE', #730, #4933, #3684 ) ;
#2860=DIRECTION ( 'NONE',  ( 5.551115123125772841E-17, -1.848892746611743135E-31, -1.000000000000000000 ) ) ;
#2867=ORIENTED_EDGE ( 'NONE', *, *, #4133, .F. ) ;
#2869=CARTESIAN_POINT ( 'NONE',  ( -84.02857808274407603, 84.45434506795682239, -11.99999999999995559 ) ) ;
#2871=EDGE_LOOP ( 'NONE', ( #2050, #221, #2588, #1314, #4510, #841, #5336, #520 ) ) ;
#2872=DIRECTION ( 'NONE',  ( -1.000000000000000000, 0.000000000000000000, 0.000000000000000000 ) ) ;
#2874=CARTESIAN_POINT ( 'NONE',  ( -84.02857808274397655, -39.54565493204319893, 152.0000000000000853 ) ) ;
#2875=CARTESIAN_POINT ( 'NONE',  ( -80.02857808274401918, 80.45434506795689344, -12.00000000000001066 ) ) ;
#2878=EDGE_CURVE ( 'NONE', #3515, #3229, #3173, .T. ) ;
#2879=ORIENTED_EDGE ( 'NONE', *, *, #4701, .T. ) ;
#2880=DIRECTION ( 'NONE',  ( -5.551115123125772841E-17, 1.848892746611743135E-31, 1.000000000000000000 ) ) ;
#2884=PLANE ( 'NONE',  #5202 ) ;
#2885=FACE_OUTER_BOUND ( 'NONE', #3774, .T. ) ;
#2889=ORIENTED_EDGE ( 'NONE', *, *, #644, .F. ) ;
#2891=DIRECTION ( 'NONE',  ( -1.000000000000000000, 0.000000000000000000, 0.000000000000000000 ) ) ;
#2894=ADVANCED_FACE ( 'NONE', ( #651 ), #1477, .T. ) ;
#2897=CARTESIAN_POINT ( 'NONE',  ( 133.9714219172562366, 80.45434506795683660, -12.00000000000001066 ) ) ;
#2908=ADVANCED_FACE ( 'NONE', ( #3194 ), #2797, .F. ) ;
#2909=ORIENTED_EDGE ( 'NONE', *, *, #5085, .T. ) ;
#2912=ADVANCED_FACE ( 'NONE', ( #4013 ), #1059, .T. ) ;
#2916=AXIS2_PLACEMENT_3D ( 'NONE', #3295, #1994, #1490 ) ;
#2920=VECTOR ( 'NONE', #2699, 1000.000000000000000 ) ;
#2926=AXIS2_PLACEMENT_3D ( 'NONE', #4646, #959, #1347 ) ;
#2927=EDGE_LOOP ( 'NONE', ( #3565, #2190, #5177, #1408 ) ) ;
#2928=LINE ( 'NONE', #1200, #1977 ) ;
#2933=EDGE_CURVE ( 'NONE', #405, #3749, #4851, .T. ) ;
#2935=AXIS2_PLACEMENT_3D ( 'NONE', #2557, #2480, #3316 ) ;
#2936=AXIS2_PLACEMENT_3D ( 'NONE', #1523, #1112, #4410 ) ;
#2944=EDGE_CURVE ( 'NONE', #2425, #483, #2714, .T. ) ;
#2948=ORIENTED_EDGE ( 'NONE', *, *, #4694, .T. ) ;
#2949=CARTESIAN_POINT ( 'NONE',  ( -77.37696704867103392, -26.07682022631158247, -10.00000000000000888 ) ) ;
#2950=DIRECTION ( 'NONE',  ( 0.4205749795070158337, 0.9072577839912276954, 0.000000000000000000 ) ) ;
#2951=LINE ( 'NONE', #857, #1699 ) ;
#2952=CARTESIAN_POINT ( 'NONE',  ( 137.9714219172561513, -25.54565493204318116, -11.99999999999995559 ) ) ;
#2956=EDGE_LOOP ( 'NONE', ( #3458, #4428, #4965, #2555, #5388, #3851, #755, #5084 ) ) ;
#2965=AXIS2_PLACEMENT_3D ( 'NONE', #4467, #3652, #1576 ) ;
#2968=CARTESIAN_POINT ( 'NONE',  ( -84.02857808274413287, 84.45434506795682239, -5.551115123125782702E-14 ) ) ;
#2969=DIRECTION ( 'NONE',  ( 1.000000000000000000, 0.000000000000000000, 0.000000000000000000 ) ) ;
#2971=VERTEX_POINT ( 'NONE', #3547 ) ;
#2974=DIRECTION ( 'NONE',  ( 5.551115123125772841E-17, -1.848892746611743135E-31, -1.000000000000000000 ) ) ;
#2975=DIRECTION ( 'NONE',  ( 5.551115123125772841E-17, -1.848892746611743135E-31, -1.000000000000000000 ) ) ;
#2976=DIRECTION ( 'NONE',  ( 1.000000000000000000, 1.261617073437686134E-16, 5.551115123125772841E-17 ) ) ;
#2977=CARTESIAN_POINT ( 'NONE',  ( 133.9714219172562366, -21.54565493204319182, -2.000000000000001776 ) ) ;
#2979=ORIENTED_EDGE ( 'NONE', *, *, #4135, .F. ) ;
#2981=EDGE_CURVE ( 'NONE', #4519, #1066, #5111, .T. ) ;
#2987=FACE_OUTER_BOUND ( 'NONE', #2257, .T. ) ;
#2988=ADVANCED_FACE ( 'NONE', ( #3661 ), #2385, .F. ) ;
#2993=DIRECTION ( 'NONE',  ( 5.551115123125772841E-17, -1.848892746611743354E-31, -1.000000000000000000 ) ) ;
#2995=ORIENTED_EDGE ( 'NONE', *, *, #2682, .T. ) ;
#2998=ADVANCED_FACE ( 'NONE', ( #5321 ), #4907, .T. ) ;
#2999=EDGE_CURVE ( 'NONE', #2650, #486, #5023, .T. ) ;
#3000=EDGE_LOOP ( 'NONE', ( #4914, #3617, #782, #2832 ) ) ;
#3002=EDGE_CURVE ( 'NONE', #964, #4350, #4369, .T. ) ;
#3003=CARTESIAN_POINT ( 'NONE',  ( -80.02857808274418971, -21.54565493204321669, -2.000000000000001776 ) ) ;
#3010=ORIENTED_EDGE ( 'NONE', *, *, #4064, .T. ) ;
#3012=AXIS2_PLACEMENT_3D ( 'NONE', #5080, #2045, #3725 ) ;
#3016=DIRECTION ( 'NONE',  ( -1.000000000000000000, 0.000000000000000000, 0.000000000000000000 ) ) ;
#3018=AXIS2_PLACEMENT_3D ( 'NONE', #299, #3954, #1531 ) ;
#3019=CIRCLE ( 'NONE', #4680, 14.00000000000002665 ) ;
#3022=ADVANCED_FACE ( 'NONE', ( #1659 ), #4969, .F. ) ;
#3024=AXIS2_PLACEMENT_3D ( 'NONE', #2446, #2860, #3707 ) ;
#3027=AXIS2_PLACEMENT_3D ( 'NONE', #1572, #1104, #5222 ) ;
#3028=VECTOR ( 'NONE', #2085, 1000.000000000000000 ) ;
#3029=ORIENTED_EDGE ( 'NONE', *, *, #3318, .T. ) ;
#3030=ORIENTED_EDGE ( 'NONE', *, *, #3479, .T. ) ;
#3031=CARTESIAN_POINT ( 'NONE',  ( -78.28422483266214726, 85.40608534173227895, -12.00000000000001066 ) ) ;
#3044=ORIENTED_EDGE ( 'NONE', *, *, #618, .T. ) ;
#3051=EDGE_LOOP ( 'NONE', ( #5273, #2205 ) ) ;
#3053=DIRECTION ( 'NONE',  ( -0.4205749795070158337, -0.9072577839912276954, 0.000000000000000000 ) ) ;
#3055=CARTESIAN_POINT ( 'NONE',  ( -82.68018911681718919, 75.92317977368848858, -12.00000000000001066 ) ) ;
#3056=ORIENTED_EDGE ( 'NONE', *, *, #3232, .T. ) ;
#3058=LINE ( 'NONE', #4346, #770 ) ;
#3060=EDGE_CURVE ( 'NONE', #1068, #339, #2841, .T. ) ;
#3063=CARTESIAN_POINT ( 'NONE',  ( -84.02857808274403340, 98.45434506795682239, -12.00000000000001066 ) ) ;
#3065=CARTESIAN_POINT ( 'NONE',  ( 132.2270686671745352, 85.40608534173219368, -11.99999999999995559 ) ) ;
#3069=VERTEX_POINT ( 'NONE', #4535 ) ;
#3070=ORIENTED_EDGE ( 'NONE', *, *, #2679, .T. ) ;
#3071=DIRECTION ( 'NONE',  ( -1.000000000000000000, 3.759415251443877379E-31, -5.551115123125772841E-17 ) ) ;
#3075=VERTEX_POINT ( 'NONE', #846 ) ;
#3076=LINE ( 'NONE', #2270, #5057 ) ;
#3079=SHAPE_REPRESENTATION ( 'Stainless Steel Outer Shield Cover', ( #2926 ), #574 ) ;
#3083=EDGE_CURVE ( 'NONE', #4995, #2687, #471, .T. ) ;
#3089=ADVANCED_FACE ( 'NONE', ( #788 ), #2884, .F. ) ;
#3091=DIRECTION ( 'NONE',  ( 0.9072577839912278064, -0.4205749795070158892, -5.551115123125773458E-17 ) ) ;
#3092=DIRECTION ( 'NONE',  ( 5.551115123125772841E-17, -1.848892746611743135E-31, -1.000000000000000000 ) ) ;
#3093=ORIENTED_EDGE ( 'NONE', *, *, #4921, .F. ) ;
#3102=CARTESIAN_POINT ( 'NONE',  ( 133.9714219172562650, 80.45434506795682239, -9.999999999999841904 ) ) ;
#3106=AXIS2_PLACEMENT_3D ( 'NONE', #4975, #2806, #1154 ) ;
#3107=AXIS2_PLACEMENT_3D ( 'NONE', #4440, #263, #2349 ) ;
#3113=VECTOR ( 'NONE', #1555, 1000.000000000000000 ) ;
#3115=EDGE_LOOP ( 'NONE', ( #1459, #4978, #4964, #5152 ) ) ;
#3117=EDGE_CURVE ( 'NONE', #3520, #1799, #3685, .T. ) ;
#3121=LINE ( 'NONE', #170, #2920 ) ;
#3127=VERTEX_POINT ( 'NONE', #2656 ) ;
#3133=CARTESIAN_POINT ( 'NONE',  ( 132.2270686671743647, -26.49739520581860575, -9.999999999999953815 ) ) ;
#3144=ORIENTED_EDGE ( 'NONE', *, *, #3232, .F. ) ;
#3145=DIRECTION ( 'NONE',  ( -2.523234146875361914E-16, -1.000000000000000000, -1.456973175402238023E-31 ) ) ;
#3150=DIRECTION ( 'NONE',  ( -2.523234146875361914E-16, -1.000000000000000000, -1.456973175402238023E-31 ) ) ;
#3152=LINE ( 'NONE', #976, #15 ) ;
#3153=ADVANCED_FACE ( 'NONE', ( #3437 ), #3841, .F. ) ;
#3154=DIRECTION ( 'NONE',  ( 5.551115123125772841E-17, -1.848892746611743354E-31, -1.000000000000000000 ) ) ;
#3156=CARTESIAN_POINT ( 'NONE',  ( -85.27857808274411866, -21.54565493204320248, -26.84924240491759662 ) ) ;
#3157=VERTEX_POINT ( 'NONE', #73 ) ;
#3158=EDGE_CURVE ( 'NONE', #3905, #5368, #453, .T. ) ;
#3159=ADVANCED_FACE ( 'NONE', ( #5125 ), #46, .F. ) ;
#3161=LINE ( 'NONE', #2196, #3325 ) ;
#3165=DIRECTION ( 'NONE',  ( -1.000000000000000000, 3.759415251443877379E-31, -5.551115123125772841E-17 ) ) ;
#3173=LINE ( 'NONE', #1070, #3979 ) ;
#3178=ORIENTED_EDGE ( 'NONE', *, *, #3496, .T. ) ;
#3183=CYLINDRICAL_SURFACE ( 'NONE', #2408, 14.00000000000004086 ) ;
#3186=CIRCLE ( 'NONE', #3536, 14.00000000000001243 ) ;
#3187=CARTESIAN_POINT ( 'NONE',  ( 132.2270686671745068, 85.40608534173219368, -9.999999999999953815 ) ) ;
#3189=EDGE_CURVE ( 'NONE', #3533, #1042, #1910, .T. ) ;
#3191=FACE_OUTER_BOUND ( 'NONE', #4462, .T. ) ;
#3192=MANIFOLD_SOLID_BREP ( 'Cut-Extrude2', #4554 ) ;
#3193=VECTOR ( 'NONE', #143, 1000.000000000000000 ) ;
#3194=FACE_OUTER_BOUND ( 'NONE', #290, .T. ) ;
#3195=AXIS2_PLACEMENT_3D ( 'NONE', #5221, #1509, #4048 ) ;
#3202=CIRCLE ( 'NONE', #1515, 5.250000000000004441 ) ;
#3207=AXIS2_PLACEMENT_3D ( 'NONE', #565, #2288, #4281 ) ;
#3212=ORIENTED_EDGE ( 'NONE', *, *, #4594, .F. ) ;
#3217=AXIS2_PLACEMENT_3D ( 'NONE', #4881, #2796, #4475 ) ;
#3218=CARTESIAN_POINT ( 'NONE',  ( -82.68018911681716077, -17.01448963777485446, -9.999999999999953815 ) ) ;
#3222=FACE_OUTER_BOUND ( 'NONE', #2871, .T. ) ;
#3223=CARTESIAN_POINT ( 'NONE',  ( -78.28422483266226095, -26.49739520581859153, -12.00000000000006573 ) ) ;
#3229=VERTEX_POINT ( 'NONE', #3598 ) ;
#3231=ORIENTED_EDGE ( 'NONE', *, *, #2419, .F. ) ;
#3232=EDGE_CURVE ( 'NONE', #4034, #4350, #1416, .T. ) ;
#3233=ADVANCED_FACE ( 'NONE', ( #2267 ), #3949, .T. ) ;
#3235=FACE_OUTER_BOUND ( 'NONE', #3115, .T. ) ;
#3238=DIRECTION ( 'NONE',  ( 5.551115123125772841E-17, -1.848892746611743135E-31, -1.000000000000000000 ) ) ;
#3257=ORIENTED_EDGE ( 'NONE', *, *, #2933, .T. ) ;
#3261=EDGE_CURVE ( 'NONE', #577, #1068, #5254, .T. ) ;
#3262=ORIENTED_EDGE ( 'NONE', *, *, #2682, .F. ) ;
#3264=ORIENTED_EDGE ( 'NONE', *, *, #2582, .T. ) ;
#3265=DIRECTION ( 'NONE',  ( -1.000000000000000000, 0.000000000000000000, 0.000000000000000000 ) ) ;
#3266=DIRECTION ( 'NONE',  ( -5.551115123125772841E-17, 1.848892746611743135E-31, 1.000000000000000000 ) ) ;
#3269=CARTESIAN_POINT ( 'NONE',  ( 133.9714219172562366, 80.45434506795683660, -12.00000000000001066 ) ) ;
#3274=CARTESIAN_POINT ( 'NONE',  ( -98.02857808274411866, 84.45434506795672291, 5.551115123125782702E-14 ) ) ;
#3277=FACE_BOUND ( 'NONE', #4489, .T. ) ;
#3281=VERTEX_POINT ( 'NONE', #3572 ) ;
#3286=CARTESIAN_POINT ( 'NONE',  ( -84.02857808274397655, -39.54565493204319893, 152.0000000000000853 ) ) ;
#3295=CARTESIAN_POINT ( 'NONE',  ( 132.2270686671745068, 85.40608534173219368, -9.999999999999953815 ) ) ;
#3296=CARTESIAN_POINT ( 'NONE',  ( -77.37696704867103392, -26.07682022631158247, -10.00000000000000888 ) ) ;
#3298=CIRCLE ( 'NONE', #3730, 5.250000000000004441 ) ;
#3299=LINE ( 'NONE', #4145, #5124 ) ;
#3301=ADVANCED_FACE ( 'NONE', ( #2289 ), #3183, .T. ) ;
#3305=DIRECTION ( 'NONE',  ( -1.000000000000000000, 3.759415251443877817E-31, -5.551115123125772841E-17 ) ) ;
#3308=DIRECTION ( 'NONE',  ( 5.551115123125772841E-17, -1.848892746611743354E-31, -1.000000000000000000 ) ) ;
#3310=CARTESIAN_POINT ( 'NONE',  ( -84.02857808274407603, -25.54565493204318116, 152.0000000000000853 ) ) ;
#3313=ORIENTED_EDGE ( 'NONE', *, *, #3501, .T. ) ;
#3316=DIRECTION ( 'NONE',  ( 1.000000000000000000, 0.000000000000000000, 0.000000000000000000 ) ) ;
#3317=ORIENTED_EDGE ( 'NONE', *, *, #5333, .T. ) ;
#3318=EDGE_CURVE ( 'NONE', #3404, #3520, #2586, .T. ) ;
#3319=PLANE ( 'NONE',  #1561 ) ;
#3320=CYLINDRICAL_SURFACE ( 'NONE', #3012, 6.000000000000032863 ) ;
#3324=CARTESIAN_POINT ( 'NONE',  ( -80.02857808274401918, 80.45434506795689344, -12.00000000000001066 ) ) ;
#3325=VECTOR ( 'NONE', #1808, 1000.000000000000000 ) ;
#3326=FACE_OUTER_BOUND ( 'NONE', #1548, .T. ) ;
#3327=CARTESIAN_POINT ( 'NONE',  ( 133.9714219172562366, -21.54565493204319182, -12.00000000000006573 ) ) ;
#3331=EDGE_CURVE ( 'NONE', #2285, #832, #881, .T. ) ;
#3337=CIRCLE ( 'NONE', #953, 6.000000000000032863 ) ;
#3342=ORIENTED_EDGE ( 'NONE', *, *, #3060, .F. ) ;
#3343=DIRECTION ( 'NONE',  ( 1.000000000000000000, 0.000000000000000000, 8.260587980841909197E-17 ) ) ;
#3347=DIRECTION ( 'NONE',  ( -1.000000000000000000, 0.000000000000000000, 0.000000000000000000 ) ) ;
#3350=FACE_OUTER_BOUND ( 'NONE', #373, .T. ) ;
#3351=CARTESIAN_POINT ( 'NONE',  ( -81.77293133282591953, -16.59391465826784540, -11.99999999999995559 ) ) ;
#3353=ADVANCED_FACE ( 'NONE', ( #4526 ), #59, .F. ) ;
#3358=FACE_OUTER_BOUND ( 'NONE', #1025, .T. ) ;
#3361=DIRECTION ( 'NONE',  ( 0.4205749795070158337, 0.9072577839912276954, 0.000000000000000000 ) ) ;
#3363=VECTOR ( 'NONE', #2259, 999.9999999999998863 ) ;
#3365=CARTESIAN_POINT ( 'NONE',  ( 137.9714219172562935, -25.54565493204318116, 152.0000000000004263 ) ) ;
#3367=CARTESIAN_POINT ( 'NONE',  ( -98.02857808274411866, 84.45434506795672291, 152.0000000000001990 ) ) ;
#3368=AXIS2_PLACEMENT_3D ( 'NONE', #4521, #3675, #3265 ) ;
#3369=DIRECTION ( 'NONE',  ( -5.551115123125772841E-17, 1.848892746611743135E-31, 1.000000000000000000 ) ) ;
#3370=DIRECTION ( 'NONE',  ( -1.000000000000000000, 3.759415251443877817E-31, -5.551115123125772841E-17 ) ) ;
#3373=ORIENTED_EDGE ( 'NONE', *, *, #2015, .T. ) ;
#3375=CIRCLE ( 'NONE', #297, 6.000000000000032863 ) ;
#3376=ORIENTED_EDGE ( 'NONE', *, *, #3158, .T. ) ;
#3378=DIRECTION ( 'NONE',  ( 5.551115123125772841E-17, -1.848892746611743135E-31, -1.000000000000000000 ) ) ;
#3380=AXIS2_PLACEMENT_3D ( 'NONE', #3487, #5114, #5168 ) ;
#3381=VECTOR ( 'NONE', #4152, 1000.000000000000000 ) ;
#3382=VECTOR ( 'NONE', #2767, 1000.000000000000000 ) ;
#3388=AXIS2_PLACEMENT_3D ( 'NONE', #982, #182, #1857 ) ;
#3390=VERTEX_POINT ( 'NONE', #1196 ) ;
#3392=AXIS2_PLACEMENT_3D ( 'NONE', #5227, #5250, #5277 ) ;
#3394=EDGE_CURVE ( 'NONE', #5106, #1160, #1996, .T. ) ;
#3396=CARTESIAN_POINT ( 'NONE',  ( 151.9714219172562650, -25.54565493204307813, -11.99999999999995559 ) ) ;
#3397=EDGE_CURVE ( 'NONE', #4488, #3530, #5051, .T. ) ;
#3399=FACE_BOUND ( 'NONE', #1047, .T. ) ;
#3402=FACE_BOUND ( 'NONE', #2202, .T. ) ;
#3403=CARTESIAN_POINT ( 'NONE',  ( -84.02857808274407603, 84.45434506795682239, -11.99999999999995559 ) ) ;
#3404=VERTEX_POINT ( 'NONE', #3701 ) ;
#3405=ORIENTED_EDGE ( 'NONE', *, *, #1301, .F. ) ;
#3406=CIRCLE ( 'NONE', #3106, 14.00000000000002665 ) ;
#3407=EDGE_LOOP ( 'NONE', ( #3950, #2603, #3443, #413, #2112, #3070, #2879, #4798 ) ) ;
#3410=CARTESIAN_POINT ( 'NONE',  ( -84.02857808274413287, 84.45434506795682239, 152.0000000000003126 ) ) ;
#3416=EDGE_CURVE ( 'NONE', #3157, #5368, #3299, .T. ) ;
#3418=ORIENTED_EDGE ( 'NONE', *, *, #3989, .F. ) ;
#3423=DIRECTION ( 'NONE',  ( -5.551115123125772841E-17, 1.848892746611743135E-31, 1.000000000000000000 ) ) ;
#3424=EDGE_CURVE ( 'NONE', #5024, #2670, #3298, .T. ) ;
#3430=EDGE_CURVE ( 'NONE', #4488, #4657, #5344, .T. ) ;
#3431=ORIENTED_EDGE ( 'NONE', *, *, #2777, .T. ) ;
#3435=LINE ( 'NONE', #3760, #2216 ) ;
#3437=FACE_OUTER_BOUND ( 'NONE', #4569, .T. ) ;
#3438=ORIENTED_EDGE ( 'NONE', *, *, #4229, .T. ) ;
#3443=ORIENTED_EDGE ( 'NONE', *, *, #4294, .T. ) ;
#3449=DIRECTION ( 'NONE',  ( -5.551115123125772841E-17, 1.848892746611743135E-31, 1.000000000000000000 ) ) ;
#3451=CARTESIAN_POINT ( 'NONE',  ( 128.7214219172562082, 80.45434506795679397, -26.84924240491753977 ) ) ;
#3452=LINE ( 'NONE', #5144, #1176 ) ;
#3453=CIRCLE ( 'NONE', #5010, 5.250000000000018652 ) ;
#3456=ORIENTED_EDGE ( 'NONE', *, *, #2777, .F. ) ;
#3457=AXIS2_PLACEMENT_3D ( 'NONE', #421, #369, #2463 ) ;
#3458=ORIENTED_EDGE ( 'NONE', *, *, #618, .F. ) ;
#3462=VECTOR ( 'NONE', #3449, 1000.000000000000000 ) ;
#3463=VECTOR ( 'NONE', #2950, 1000.000000000000114 ) ;
#3465=ORIENTED_EDGE ( 'NONE', *, *, #4823, .T. ) ;
#3477=STYLED_ITEM('',(#5458),#1341);
#3479=EDGE_CURVE ( 'NONE', #3520, #3404, #1877, .T. ) ;
#3480=ORIENTED_EDGE ( 'NONE', *, *, #3989, .T. ) ;
#3483=LINE ( 'NONE', #62, #723 ) ;
#3484=LINE ( 'NONE', #2142, #4863 ) ;
#3486=LINE ( 'NONE', #5143, #1677 ) ;
#3487=CARTESIAN_POINT ( 'NONE',  ( -84.02857808274418971, -25.54565493204318116, -5.551115123125782702E-14 ) ) ;
#3488=ORIENTED_EDGE ( 'NONE', *, *, #1935, .T. ) ;
#3496=EDGE_CURVE ( 'NONE', #2476, #1072, #4271, .T. ) ;
#3498=CYLINDRICAL_SURFACE ( 'NONE', #4603, 6.000000000000032863 ) ;
#3501=EDGE_CURVE ( 'NONE', #3639, #339, #3782, .T. ) ;
#3507=EDGE_CURVE ( 'NONE', #3530, #3127, #3553, .T. ) ;
#3515=VERTEX_POINT ( 'NONE', #933 ) ;
#3516=ORIENTED_EDGE ( 'NONE', *, *, #3397, .T. ) ;
#3518=DIRECTION ( 'NONE',  ( -1.000000000000000000, 0.000000000000000000, 0.000000000000000000 ) ) ;
#3520=VERTEX_POINT ( 'NONE', #4588 ) ;
#3523=CARTESIAN_POINT ( 'NONE',  ( 136.6230329513293498, 75.92317977368846016, -11.99999999999995559 ) ) ;
#3530=VERTEX_POINT ( 'NONE', #434 ) ;
#3533=VERTEX_POINT ( 'NONE', #2614 ) ;
#3536=AXIS2_PLACEMENT_3D ( 'NONE', #4581, #1278, #3807 ) ;
#3542=DIRECTION ( 'NONE',  ( -1.000000000000000000, 0.000000000000000000, 0.000000000000000000 ) ) ;
#3547=CARTESIAN_POINT ( 'NONE',  ( 135.7157751673381085, -16.59391465826787027, -9.999999999999953815 ) ) ;
#3552=AXIS2_PLACEMENT_3D ( 'NONE', #3919, #145, #4758 ) ;
#3553=CIRCLE ( 'NONE', #1440, 14.00000000000004086 ) ;
#3560=ADVANCED_FACE ( 'NONE', ( #1283 ), #518, .F. ) ;
#3563=EDGE_CURVE ( 'NONE', #2642, #2780, #3484, .T. ) ;
#3564=EDGE_CURVE ( 'NONE', #1930, #3639, #4691, .T. ) ;
#3565=ORIENTED_EDGE ( 'NONE', *, *, #4623, .T. ) ;
#3568=CARTESIAN_POINT ( 'NONE',  ( 151.9714219172562935, 84.45434506795673713, -11.99999999999995559 ) ) ;
#3570=DIRECTION ( 'NONE',  ( 5.551115123125772841E-17, -1.848892746611743135E-31, -1.000000000000000000 ) ) ;
#3571=FACE_OUTER_BOUND ( 'NONE', #4807, .T. ) ;
#3572=CARTESIAN_POINT ( 'NONE',  ( -86.02857808274413287, -21.54565493204320248, -12.00000000000001066 ) ) ;
#3577=DIRECTION ( 'NONE',  ( 0.4205749795070158337, 0.9072577839912276954, 0.000000000000000000 ) ) ;
#3586=ORIENTED_EDGE ( 'NONE', *, *, #3858, .F. ) ;
#3587=CARTESIAN_POINT ( 'NONE',  ( 132.2270686671745068, 85.40608534173219368, -9.999999999999953815 ) ) ;
#3590=UNCERTAINTY_MEASURE_WITH_UNIT (LENGTH_MEASURE( 1.000000000000000082E-05 ), #5203, 'distance_accuracy_value', 'NONE');
#3592=LINE ( 'NONE', #1467, #1254 ) ;
#3593=CARTESIAN_POINT ( 'NONE',  ( 133.9714219172562650, 80.45434506795683660, -2.000000000000001776 ) ) ;
#3596=FACE_OUTER_BOUND ( 'NONE', #5409, .T. ) ;
#3597=ADVANCED_FACE ( 'NONE', ( #3358 ), #1313, .T. ) ;
#3598=CARTESIAN_POINT ( 'NONE',  ( -81.77293133282584847, 75.50260479418152215, -11.99999999999995559 ) ) ;
#3617=ORIENTED_EDGE ( 'NONE', *, *, #2774, .F. ) ;
#3618=LINE ( 'NONE', #1551, #382 ) ;
#3621=LINE ( 'NONE', #1603, #1887 ) ;
#3622=EDGE_LOOP ( 'NONE', ( #654, #1024, #4834, #1363 ) ) ;
#3624=DIRECTION ( 'NONE',  ( 5.551115123125772841E-17, -1.848892746611743354E-31, -1.000000000000000000 ) ) ;
#3628=CIRCLE ( 'NONE', #985, 5.250000000000004441 ) ;
#3630=CARTESIAN_POINT ( 'NONE',  ( -80.02857808274418971, -21.54565493204321669, -2.000000000000001776 ) ) ;
#3631=EDGE_CURVE ( 'NONE', #1799, #783, #1087, .T. ) ;
#3632=VECTOR ( 'NONE', #1758, 999.9999999999998863 ) ;
#3638=AXIS2_PLACEMENT_3D ( 'NONE', #1892, #2275, #2734 ) ;
#3639=VERTEX_POINT ( 'NONE', #849 ) ;
#3641=ORIENTED_EDGE ( 'NONE', *, *, #3424, .F. ) ;
#3642=CARTESIAN_POINT ( 'NONE',  ( -78.28422483266231779, -26.49739520581859153, -10.00000000000006395 ) ) ;
#3644=LINE ( 'NONE', #5306, #2847 ) ;
#3645=CIRCLE ( 'NONE', #1344, 6.000000000000032863 ) ;
#3647=UNCERTAINTY_MEASURE_WITH_UNIT (LENGTH_MEASURE( 1.000000000000000082E-05 ), #4930, 'distance_accuracy_value', 'NONE');
#3648=VECTOR ( 'NONE', #4241, 1000.000000000000000 ) ;
#3649=CIRCLE ( 'NONE', #1798, 5.250000000000018652 ) ;
#3651=DIRECTION ( 'NONE',  ( 5.551115123125772841E-17, -1.848892746611743135E-31, -1.000000000000000000 ) ) ;
#3652=DIRECTION ( 'NONE',  ( 5.551115123125772841E-17, -1.848892746611743135E-31, -1.000000000000000000 ) ) ;
#3654=PLANE ( 'NONE',  #4074 ) ;
#3655=CIRCLE ( 'NONE', #131, 6.000000000000032863 ) ;
#3656=DIRECTION ( 'NONE',  ( 3.204747427460360459E-31, -1.000000000000000000, 1.848892746611743354E-31 ) ) ;
#3658=DIRECTION ( 'NONE',  ( 5.551115123125772841E-17, -1.848892746611743135E-31, -1.000000000000000000 ) ) ;
#3660=PLANE ( 'NONE',  #2855 ) ;
#3661=FACE_OUTER_BOUND ( 'NONE', #5413, .T. ) ;
#3666=EDGE_CURVE ( 'NONE', #405, #3533, #2501, .T. ) ;
#3667=ADVANCED_FACE ( 'NONE', ( #1810 ), #3498, .F. ) ;
#3668=ORIENTED_EDGE ( 'NONE', *, *, #3501, .F. ) ;
#3670=VECTOR ( 'NONE', #5305, 1000.000000000000000 ) ;
#3671=ORIENTED_EDGE ( 'NONE', *, *, #1674, .T. ) ;
#3673=EDGE_LOOP ( 'NONE', ( #4411, #3480, #4928 ) ) ;
#3675=DIRECTION ( 'NONE',  ( 5.551115123125772841E-17, -1.848892746611743135E-31, -1.000000000000000000 ) ) ;
#3678=CARTESIAN_POINT ( 'NONE',  ( -80.02857808274404761, 80.45434506795689344, -9.999999999999841904 ) ) ;
#3679=DIRECTION ( 'NONE',  ( 5.551115123125772841E-17, -1.848892746611743135E-31, -1.000000000000000000 ) ) ;
#3682=CARTESIAN_POINT ( 'NONE',  ( -85.27857808274414708, 80.45434506795689344, -26.84924240491753977 ) ) ;
#3684=DIRECTION ( 'NONE',  ( -1.000000000000000000, 3.759415251443877379E-31, -5.551115123125772841E-17 ) ) ;
#3685=LINE ( 'NONE', #1205, #3381 ) ;
#3687=EDGE_CURVE ( 'NONE', #4708, #484, #4012, .T. ) ;
#3692=VERTEX_POINT ( 'NONE', #3055 ) ;
#3696=ORIENTED_EDGE ( 'NONE', *, *, #4133, .T. ) ;
#3697=CYLINDRICAL_SURFACE ( 'NONE', #3895, 14.00000000000001243 ) ;
#3699=CARTESIAN_POINT ( 'NONE',  ( 131.3198108831832656, 84.98551036222518462, -10.00000000000000888 ) ) ;
#3700=CARTESIAN_POINT ( 'NONE',  ( 151.9714219172563219, 84.45434506795673713, 152.0000000000001990 ) ) ;
#3701=CARTESIAN_POINT ( 'NONE',  ( 139.9714219172562935, 80.45434506795683660, -2.000000000000001332 ) ) ;
#3707=DIRECTION ( 'NONE',  ( -1.000000000000000000, 0.000000000000000000, -7.228014483236656373E-17 ) ) ;
#3708=CARTESIAN_POINT ( 'NONE',  ( -86.02857808274404761, 80.45434506795689344, -2.000000000000113243 ) ) ;
#3714=AXIS2_PLACEMENT_3D ( 'NONE', #2952, #3369, #33 ) ;
#3717=VECTOR ( 'NONE', #4437, 1000.000000000000000 ) ;
#3721=EDGE_CURVE ( 'NONE', #3127, #979, #5132, .T. ) ;
#3725=DIRECTION ( 'NONE',  ( -1.000000000000000000, 0.000000000000000000, -7.228014483236656373E-17 ) ) ;
#3726=CARTESIAN_POINT ( 'NONE',  ( -77.37696704867103392, 84.98551036222526989, -11.99999999999990052 ) ) ;
#3729=EDGE_CURVE ( 'NONE', #265, #1569, #241, .T. ) ;
#3730=AXIS2_PLACEMENT_3D ( 'NONE', #3269, #3679, #5367 ) ;
#3731=AXIS2_PLACEMENT_3D ( 'NONE', #4846, #672, #4122 ) ;
#3734=ORIENTED_EDGE ( 'NONE', *, *, #3261, .F. ) ;
#3735=CARTESIAN_POINT ( 'NONE',  ( 139.9714219172562650, 80.45434506795683660, -12.00000000000001066 ) ) ;
#3738=DIRECTION ( 'NONE',  ( 1.000000000000000000, 0.000000000000000000, 8.260587980841931384E-17 ) ) ;
#3740=DIRECTION ( 'NONE',  ( 5.551115123125772841E-17, -1.848892746611743135E-31, -1.000000000000000000 ) ) ;
#3741=PRODUCT_DEFINITION_FORMATION_WITH_SPECIFIED_SOURCE ( 'ANY', '', #1704, .NOT_KNOWN. ) ;
#3746=EDGE_CURVE ( 'NONE', #496, #1327, #5389, .T. ) ;
#3748=CARTESIAN_POINT ( 'NONE',  ( 128.7214219172562366, 80.45434506795679397, -12.00000000000001066 ) ) ;
#3749=VERTEX_POINT ( 'NONE', #3523 ) ;
#3750=EDGE_LOOP ( 'NONE', ( #359, #2569 ) ) ;
#3751=DIRECTION ( 'NONE',  ( 5.551115123125772841E-17, -1.848892746611743135E-31, -1.000000000000000000 ) ) ;
#3760=CARTESIAN_POINT ( 'NONE',  ( 139.9714219172563219, 80.45434506795683660, -2.000000000000001332 ) ) ;
#3761=DIRECTION ( 'NONE',  ( 2.523234146875361914E-16, 1.000000000000000000, 1.456973175402238023E-31 ) ) ;
#3765=CARTESIAN_POINT ( 'NONE',  ( -77.37696704867103392, -26.07682022631158247, -10.00000000000000888 ) ) ;
#3766=VERTEX_POINT ( 'NONE', #5180 ) ;
#3768=DIRECTION ( 'NONE',  ( -1.000000000000000000, 0.000000000000000000, 0.000000000000000000 ) ) ;
#3770=CARTESIAN_POINT ( 'NONE',  ( 133.9714219172562366, -21.54565493204319182, -12.00000000000006573 ) ) ;
#3774=EDGE_LOOP ( 'NONE', ( #2703, #393, #1766, #3516, #5187, #4095, #3696, #2830 ) ) ;
#3775=EDGE_LOOP ( 'NONE', ( #4357, #930, #4382, #688 ) ) ;
#3777=DIRECTION ( 'NONE',  ( -1.000000000000000000, 0.000000000000000000, 0.000000000000000000 ) ) ;
#3782=LINE ( 'NONE', #50, #3028 ) ;
#3785=ORIENTED_EDGE ( 'NONE', *, *, #2482, .F. ) ;
#3786=ORIENTED_EDGE ( 'NONE', *, *, #3416, .T. ) ;
#3792=CARTESIAN_POINT ( 'NONE',  ( 137.9714219172560945, -39.54565493204318471, -11.99999999999995559 ) ) ;
#3799=ADVANCED_FACE ( 'NONE', ( #3902 ), #1891, .F. ) ;
#3804=EDGE_CURVE ( 'NONE', #994, #1569, #919, .T. ) ;
#3807=DIRECTION ( 'NONE',  ( 1.000000000000000000, 0.000000000000000000, 0.000000000000000000 ) ) ;
#3813=ORIENTED_EDGE ( 'NONE', *, *, #4780, .T. ) ;
#3814=VECTOR ( 'NONE', #1318, 1000.000000000000000 ) ;
#3815=AXIS2_PLACEMENT_3D ( 'NONE', #868, #2572, #3738 ) ;
#3819=DIRECTION ( 'NONE',  ( 5.551115123125772841E-17, -1.848892746611743135E-31, -1.000000000000000000 ) ) ;
#3829=ORIENTED_EDGE ( 'NONE', *, *, #5085, .F. ) ;
#3831=CARTESIAN_POINT ( 'NONE',  ( 131.3198108831832371, 84.98551036222518462, -11.99999999999995559 ) ) ;
#3833=CYLINDRICAL_SURFACE ( 'NONE', #3714, 14.00000000000001243 ) ;
#3836=ORIENTED_EDGE ( 'NONE', *, *, #2482, .T. ) ;
#3841=CYLINDRICAL_SURFACE ( 'NONE', #2401, 6.000000000000032863 ) ;
#3851=ORIENTED_EDGE ( 'NONE', *, *, #795, .F. ) ;
#3853=ORIENTED_EDGE ( 'NONE', *, *, #1776, .F. ) ;
#3854=LINE ( 'NONE', #4624, #1781 ) ;
#3858=EDGE_CURVE ( 'NONE', #534, #179, #3655, .T. ) ;
#3861=ORIENTED_EDGE ( 'NONE', *, *, #2435, .T. ) ;
#3862=CARTESIAN_POINT ( 'NONE',  ( -84.02857808274400497, -39.54565493204319893, -11.99999999999984368 ) ) ;
#3864=DIRECTION ( 'NONE',  ( 5.551115123125772841E-17, -1.848892746611743135E-31, -1.000000000000000000 ) ) ;
#3866=ORIENTED_EDGE ( 'NONE', *, *, #13, .T. ) ;
#3868=EDGE_CURVE ( 'NONE', #1042, #2670, #2471, .T. ) ;
#3871=CARTESIAN_POINT ( 'NONE',  ( 133.9714219172562366, 80.45434506795683660, -12.00000000000001066 ) ) ;
#3874=CARTESIAN_POINT ( 'NONE',  ( -86.02857808274404761, 80.45434506795689344, -12.00000000000001066 ) ) ;
#3877=AXIS2_PLACEMENT_3D ( 'NONE', #1396, #5173, #2218 ) ;
#3878=CARTESIAN_POINT ( 'NONE',  ( -85.27857808274403340, 80.45434506795689344, -12.00000000000001066 ) ) ;
#3882=AXIS2_PLACEMENT_3D ( 'NONE', #2977, #5394, #2488 ) ;
#3883=ORIENTED_EDGE ( 'NONE', *, *, #2813, .T. ) ;
#3887=EDGE_CURVE ( 'NONE', #3127, #2337, #296, .T. ) ;
#3891=CARTESIAN_POINT ( 'NONE',  ( -77.37696704867111919, -26.07682022631158247, -11.99999999999995559 ) ) ;
#3895=AXIS2_PLACEMENT_3D ( 'NONE', #3365, #2975, #2872 ) ;
#3897=EDGE_LOOP ( 'NONE', ( #3734, #4221, #2490, #4894, #4548, #2037, #3313, #1598 ) ) ;
#3902=FACE_OUTER_BOUND ( 'NONE', #4426, .T. ) ;
#3904=AXIS2_PLACEMENT_3D ( 'NONE', #4441, #670, #348 ) ;
#3905=VERTEX_POINT ( 'NONE', #3274 ) ;
#3907=VECTOR ( 'NONE', #5385, 1000.000000000000000 ) ;
#3910=AXIS2_PLACEMENT_3D ( 'NONE', #3327, #811, #3016 ) ;
#3911=AXIS2_PLACEMENT_3D ( 'NONE', #2264, #1741, #3071 ) ;
#3916=ADVANCED_FACE ( 'NONE', ( #3191 ), #3660, .T. ) ;
#3917=FACE_OUTER_BOUND ( 'NONE', #5307, .T. ) ;
#3918=CARTESIAN_POINT ( 'NONE',  ( 132.2270686671743647, -26.49739520581860575, -9.999999999999953815 ) ) ;
#3919=CARTESIAN_POINT ( 'NONE',  ( -84.02857808274410445, -25.54565493204318116, -11.99999999999995559 ) ) ;
#3920=AXIS2_PLACEMENT_3D ( 'NONE', #5346, #3624, #5284 ) ;
#3923=UNCERTAINTY_MEASURE_WITH_UNIT (LENGTH_MEASURE( 1.000000000000000082E-05 ), #5102, 'distance_accuracy_value', 'NONE');
#3924=ORIENTED_EDGE ( 'NONE', *, *, #4630, .T. ) ;
#3931=CYLINDRICAL_SURFACE ( 'NONE', #1726, 6.000000000000032863 ) ;
#3933=CARTESIAN_POINT ( 'NONE',  ( -74.77857808274411866, 80.45434506795689344, -26.84924240491753977 ) ) ;
#3934=CARTESIAN_POINT ( 'NONE',  ( 137.9714219172562650, 84.45434506795687923, -5.551115123125782702E-14 ) ) ;
#3936=CIRCLE ( 'NONE', #5063, 14.00000000000004086 ) ;
#3946=PLANE ( 'NONE',  #3911 ) ;
#3949=CYLINDRICAL_SURFACE ( 'NONE', #2936, 5.250000000000004441 ) ;
#3950=ORIENTED_EDGE ( 'NONE', *, *, #3083, .T. ) ;
#3951=CARTESIAN_POINT ( 'NONE',  ( 131.3198108831832656, 84.98551036222518462, -10.00000000000000888 ) ) ;
#3954=DIRECTION ( 'NONE',  ( 5.551115123125772841E-17, -1.848892746611743135E-31, -1.000000000000000000 ) ) ;
#3956=ADVANCED_FACE ( 'NONE', ( #3222 ), #4532, .F. ) ;
#3959=EDGE_CURVE ( 'NONE', #4657, #167, #2384, .T. ) ;
#3960=EDGE_CURVE ( 'NONE', #1072, #832, #1883, .T. ) ;
#3964=FACE_OUTER_BOUND ( 'NONE', #3897, .T. ) ;
#3970=CARTESIAN_POINT ( 'NONE',  ( 137.9714219172562366, 84.45434506795687923, -12.00000000000001066 ) ) ;
#3972=ORIENTED_EDGE ( 'NONE', *, *, #2878, .F. ) ;
#3974=EDGE_CURVE ( 'NONE', #4519, #2521, #1637, .T. ) ;
#3979=VECTOR ( 'NONE', #662, 1000.000000000000000 ) ;
#3981=DIRECTION ( 'NONE',  ( 5.551115123125772841E-17, -1.848892746611743135E-31, -1.000000000000000000 ) ) ;
#3982=CIRCLE ( 'NONE', #1612, 14.00000000000002665 ) ;
#3989=EDGE_CURVE ( 'NONE', #4465, #2285, #2677, .T. ) ;
#3991=ORIENTED_EDGE ( 'NONE', *, *, #3666, .T. ) ;
#4002=ORIENTED_EDGE ( 'NONE', *, *, #2182, .T. ) ;
#4003=LINE ( 'NONE', #4027, #2133 ) ;
#4004=CARTESIAN_POINT ( 'NONE',  ( -86.02857808274421814, -21.54565493204321669, -2.000000000000002220 ) ) ;
#4005=LINE ( 'NONE', #3699, #1071 ) ;
#4007=DIRECTION ( 'NONE',  ( 5.551115123125772841E-17, -1.848892746611743135E-31, -1.000000000000000000 ) ) ;
#4008=ORIENTED_EDGE ( 'NONE', *, *, #2981, .T. ) ;
#4009=PLANE ( 'NONE',  #3920 ) ;
#4012=LINE ( 'NONE', #1420, #827 ) ;
#4013=FACE_OUTER_BOUND ( 'NONE', #141, .T. ) ;
#4014=FACE_OUTER_BOUND ( 'NONE', #4400, .T. ) ;
#4018=EDGE_LOOP ( 'NONE', ( #747, #3144, #4896, #1100 ) ) ;
#4021=DIRECTION ( 'NONE',  ( 1.000000000000000000, 0.000000000000000000, 0.000000000000000000 ) ) ;
#4025=ORIENTED_EDGE ( 'NONE', *, *, #3868, .T. ) ;
#4026=ORIENTED_EDGE ( 'NONE', *, *, #531, .F. ) ;
#4027=CARTESIAN_POINT ( 'NONE',  ( 131.3198108831832087, -26.07682022631159668, -10.00000000000000888 ) ) ;
#4030=DIRECTION ( 'NONE',  ( -1.000000000000000000, -3.125627884642856345E-17, -5.551115123125772841E-17 ) ) ;
#4032=ADVANCED_FACE ( 'NONE', ( #2987 ), #4661, .F. ) ;
#4034=VERTEX_POINT ( 'NONE', #2495 ) ;
#4035=CARTESIAN_POINT ( 'NONE',  ( -84.02857808274403340, 98.45434506795682239, -5.551115123125782702E-14 ) ) ;
#4037=CARTESIAN_POINT ( 'NONE',  ( -84.02857808274410445, -25.54565493204318116, -11.99999999999995559 ) ) ;
#4039=PLANE ( 'NONE',  #4291 ) ;
#4048=DIRECTION ( 'NONE',  ( 1.000000000000000000, 0.000000000000000000, 0.000000000000000000 ) ) ;
#4054=DIRECTION ( 'NONE',  ( -1.000000000000000000, 0.000000000000000000, -8.260587980841931384E-17 ) ) ;
#4056=DIRECTION ( 'NONE',  ( -1.000000000000000000, 0.000000000000000000, 0.000000000000000000 ) ) ;
#4062=( NAMED_UNIT ( * ) SI_UNIT ( $, .STERADIAN. ) SOLID_ANGLE_UNIT ( ) );
#4064=EDGE_CURVE ( 'NONE', #2337, #664, #4180, .T. ) ;
#4074=AXIS2_PLACEMENT_3D ( 'NONE', #3678, #4524, #5314 ) ;
#4076=ORIENTED_EDGE ( 'NONE', *, *, #2999, .F. ) ;
#4080=CIRCLE ( 'NONE', #4598, 6.000000000000032863 ) ;
#4088=DIRECTION ( 'NONE',  ( -5.551115123125772841E-17, 1.848892746611743135E-31, 1.000000000000000000 ) ) ;
#4093=CIRCLE ( 'NONE', #3392, 5.250000000000018652 ) ;
#4095=ORIENTED_EDGE ( 'NONE', *, *, #3887, .T. ) ;
#4098=CYLINDRICAL_SURFACE ( 'NONE', #3731, 6.000000000000032863 ) ;
#4101=VECTOR ( 'NONE', #4819, 1000.000000000000000 ) ;
#4103=DIRECTION ( 'NONE',  ( 1.000000000000000000, 0.000000000000000000, 7.228014483236656373E-17 ) ) ;
#4106=ORIENTED_EDGE ( 'NONE', *, *, #2854, .T. ) ;
#4114=DIRECTION ( 'NONE',  ( -0.4205749795070158337, -0.9072577839912276954, 0.000000000000000000 ) ) ;
#4116=DIRECTION ( 'NONE',  ( 5.551115123125772841E-17, -1.848892746611743135E-31, -1.000000000000000000 ) ) ;
#4117=DIRECTION ( 'NONE',  ( 5.551115123125772841E-17, -1.848892746611743135E-31, -1.000000000000000000 ) ) ;
#4122=DIRECTION ( 'NONE',  ( -1.000000000000000000, 0.000000000000000000, -7.228014483236656373E-17 ) ) ;
#4133=EDGE_CURVE ( 'NONE', #2337, #850, #4430, .T. ) ;
#4134=DIRECTION ( 'NONE',  ( -0.4205749795070158337, -0.9072577839912276954, 0.000000000000000000 ) ) ;
#4135=EDGE_CURVE ( 'NONE', #4528, #265, #4265, .T. ) ;
#4139=DIRECTION ( 'NONE',  ( 5.551115123125772841E-17, -1.848892746611743135E-31, -1.000000000000000000 ) ) ;
#4141=PLANE ( 'NONE',  #3882 ) ;
#4145=CARTESIAN_POINT ( 'NONE',  ( -98.02857808274420393, -25.54565493204307813, 152.0000000000001990 ) ) ;
#4146=ORIENTED_EDGE ( 'NONE', *, *, #3261, .T. ) ;
#4147=ORIENTED_EDGE ( 'NONE', *, *, #4457, .F. ) ;
#4149=CARTESIAN_POINT ( 'NONE',  ( -77.37696704867103392, 84.98551036222526989, -11.99999999999990052 ) ) ;
#4152=DIRECTION ( 'NONE',  ( 5.551115123125772841E-17, -1.848892746611743135E-31, -1.000000000000000000 ) ) ;
#4158=AXIS2_PLACEMENT_3D ( 'NONE', #234, #1078, #1553 ) ;
#4166=VECTOR ( 'NONE', #96, 1000.000000000000000 ) ;
#4167=DIRECTION ( 'NONE',  ( -1.000000000000000000, 0.000000000000000000, 0.000000000000000000 ) ) ;
#4172=AXIS2_PLACEMENT_3D ( 'NONE', #3871, #4264, #5097 ) ;
#4173=ORIENTED_EDGE ( 'NONE', *, *, #2417, .T. ) ;
#4180=LINE ( 'NONE', #72, #2149 ) ;
#4184=DIRECTION ( 'NONE',  ( -5.551115123125772841E-17, 1.848892746611743135E-31, 1.000000000000000000 ) ) ;
#4187=ADVANCED_FACE ( 'NONE', ( #1882 ), #2632, .F. ) ;
#4193=LINE ( 'NONE', #1672, #389 ) ;
#4195=VERTEX_POINT ( 'NONE', #4361 ) ;
#4199=EDGE_CURVE ( 'NONE', #4710, #1493, #2219, .T. ) ;
#4200=CIRCLE ( 'NONE', #1562, 5.250000000000004441 ) ;
#4211=DIRECTION ( 'NONE',  ( -5.551115123125772841E-17, 1.848892746611743135E-31, 1.000000000000000000 ) ) ;
#4217=CARTESIAN_POINT ( 'NONE',  ( 151.9714219172562650, -25.54565493204307813, -11.99999999999995559 ) ) ;
#4218=VERTEX_POINT ( 'NONE', #2655 ) ;
#4221=ORIENTED_EDGE ( 'NONE', *, *, #2344, .F. ) ;
#4222=DIRECTION ( 'NONE',  ( -5.551115123125772841E-17, 1.848892746611743354E-31, 1.000000000000000000 ) ) ;
#4229=EDGE_CURVE ( 'NONE', #1493, #556, #996, .T. ) ;
#4233=CARTESIAN_POINT ( 'NONE',  ( -80.02857808274410445, -21.54565493204320248, -12.00000000000001066 ) ) ;
#4236=VERTEX_POINT ( 'NONE', #150 ) ;
#4238=DIRECTION ( 'NONE',  ( 5.551115123125772841E-17, -1.848892746611743135E-31, -1.000000000000000000 ) ) ;
#4241=DIRECTION ( 'NONE',  ( 2.523234146875361914E-16, 1.000000000000000000, 1.456973175402238023E-31 ) ) ;
#4245=DIRECTION ( 'NONE',  ( 5.551115123125772841E-17, -1.848892746611743135E-31, -1.000000000000000000 ) ) ;
#4246=PLANE ( 'NONE',  #2153 ) ;
#4249=ORIENTED_EDGE ( 'NONE', *, *, #3960, .F. ) ;
#4250=VECTOR ( 'NONE', #1744, 1000.000000000000000 ) ;
#4252=FACE_BOUND ( 'NONE', #5100, .T. ) ;
#4253=CYLINDRICAL_SURFACE ( 'NONE', #4406, 5.250000000000018652 ) ;
#4264=DIRECTION ( 'NONE',  ( 5.551115123125772841E-17, -1.848892746611743135E-31, -1.000000000000000000 ) ) ;
#4265=CIRCLE ( 'NONE', #4683, 5.250000000000018652 ) ;
#4271=LINE ( 'NONE', #2850, #1690 ) ;
#4272=LINE ( 'NONE', #855, #1343 ) ;
#4280=DIRECTION ( 'NONE',  ( 1.000000000000000000, 0.000000000000000000, 0.000000000000000000 ) ) ;
#4281=DIRECTION ( 'NONE',  ( 1.000000000000000000, 0.000000000000000000, 0.000000000000000000 ) ) ;
#4282=DIRECTION ( 'NONE',  ( 5.551115123125772841E-17, -1.848892746611743135E-31, -1.000000000000000000 ) ) ;
#4284=AXIS2_PLACEMENT_3D ( 'NONE', #3102, #2711, #2688 ) ;
#4289=ORIENTED_EDGE ( 'NONE', *, *, #422, .T. ) ;
#4290=ORIENTED_EDGE ( 'NONE', *, *, #3974, .F. ) ;
#4291=AXIS2_PLACEMENT_3D ( 'NONE', #1980, #4501, #2449 ) ;
#4293=ADVANCED_FACE ( 'NONE', ( #3571 ), #5230, .T. ) ;
#4294=EDGE_CURVE ( 'NONE', #4195, #5106, #3982, .T. ) ;
#4295=ORIENTED_EDGE ( 'NONE', *, *, #4457, .T. ) ;
#4300=CARTESIAN_POINT ( 'NONE',  ( -98.02857808274420393, -25.54565493204309234, 5.551115123125782702E-14 ) ) ;
#4315=DIRECTION ( 'NONE',  ( -5.551115123125772841E-17, 1.848892746611743135E-31, 1.000000000000000000 ) ) ;
#4322=ADVANCED_FACE ( 'NONE', ( #3596 ), #347, .T. ) ;
#4325=DIRECTION ( 'NONE',  ( -1.000000000000000000, -3.125627884642856345E-17, -5.551115123125772841E-17 ) ) ;
#4327=DIRECTION ( 'NONE',  ( -2.523234146875361914E-16, -1.000000000000000000, -1.456973175402238023E-31 ) ) ;
#4330=VERTEX_POINT ( 'NONE', #3296 ) ;
#4338=PLANE ( 'NONE',  #4284 ) ;
#4346=CARTESIAN_POINT ( 'NONE',  ( 137.9714219172561798, 98.45434506795687923, -5.551115123125782702E-14 ) ) ;
#4350=VERTEX_POINT ( 'NONE', #2320 ) ;
#4352=ORIENTED_EDGE ( 'NONE', *, *, #3117, .T. ) ;
#4353=CARTESIAN_POINT ( 'NONE',  ( 133.9714219172562366, 80.45434506795683660, -12.00000000000001066 ) ) ;
#4357=ORIENTED_EDGE ( 'NONE', *, *, #2519, .T. ) ;
#4361=CARTESIAN_POINT ( 'NONE',  ( 137.9714219172561513, 98.45434506795689344, -12.00000000000006573 ) ) ;
#4362=ORIENTED_EDGE ( 'NONE', *, *, #422, .F. ) ;
#4363=EDGE_CURVE ( 'NONE', #2285, #800, #219, .T. ) ;
#4364=ADVANCED_FACE ( 'NONE', ( #4409 ), #3654, .T. ) ;
#4365=CARTESIAN_POINT ( 'NONE',  ( -78.28422483266214726, 85.40608534173227895, -12.00000000000001066 ) ) ;
#4366=EDGE_CURVE ( 'NONE', #3530, #167, #669, .T. ) ;
#4368=CARTESIAN_POINT ( 'NONE',  ( 133.9714219172562650, 80.45434506795683660, -2.000000000000001776 ) ) ;
#4369=LINE ( 'NONE', #3223, #1962 ) ;
#4375=ORIENTED_EDGE ( 'NONE', *, *, #3331, .F. ) ;
#4382=ORIENTED_EDGE ( 'NONE', *, *, #1870, .F. ) ;
#4383=CARTESIAN_POINT ( 'NONE',  ( -78.28422483266226095, -26.49739520581859153, -12.00000000000006573 ) ) ;
#4387=ORIENTED_EDGE ( 'NONE', *, *, #2540, .T. ) ;
#4388=CARTESIAN_POINT ( 'NONE',  ( 139.2214219172562935, 80.45434506795679397, -2.000000000000001332 ) ) ;
#4392=CARTESIAN_POINT ( 'NONE',  ( -84.02857808274407603, 84.45434506795682239, -11.99999999999995559 ) ) ;
#4393=EDGE_CURVE ( 'NONE', #2228, #2627, #3621, .T. ) ;
#4400=EDGE_LOOP ( 'NONE', ( #2316, #1000, #435, #3924 ) ) ;
#4401=DIRECTION ( 'NONE',  ( -1.000000000000000000, 2.523234146875361914E-16, -5.551115123125772841E-17 ) ) ;
#4404=VERTEX_POINT ( 'NONE', #1908 ) ;
#4406=AXIS2_PLACEMENT_3D ( 'NONE', #5402, #5090, #1331 ) ;
#4409=FACE_OUTER_BOUND ( 'NONE', #4663, .T. ) ;
#4410=DIRECTION ( 'NONE',  ( 1.000000000000000000, 0.000000000000000000, 0.000000000000000000 ) ) ;
#4411=ORIENTED_EDGE ( 'NONE', *, *, #5428, .F. ) ;
#4412=CIRCLE ( 'NONE', #4158, 14.00000000000002665 ) ;
#4416=VECTOR ( 'NONE', #242, 1000.000000000000000 ) ;
#4418=DIRECTION ( 'NONE',  ( 1.000000000000000000, 0.000000000000000000, 0.000000000000000000 ) ) ;
#4426=EDGE_LOOP ( 'NONE', ( #991, #3972, #5225, #1197 ) ) ;
#4428=ORIENTED_EDGE ( 'NONE', *, *, #1935, .F. ) ;
#4429=ADVANCED_FACE ( 'NONE', ( #1166 ), #4960, .T. ) ;
#4430=CIRCLE ( 'NONE', #1092, 14.00000000000002665 ) ;
#4432=ADVANCED_BREP_SHAPE_REPRESENTATION ( '', ( #1341, #3192, #2926 ), #574 ) ;
#4436=ORIENTED_EDGE ( 'NONE', *, *, #3397, .F. ) ;
#4437=DIRECTION ( 'NONE',  ( -1.000000000000000000, -3.125627884642856345E-17, -5.551115123125772841E-17 ) ) ;
#4440=CARTESIAN_POINT ( 'NONE',  ( -98.02857808274411866, 84.45434506795672291, -12.00000000000001066 ) ) ;
#4441=CARTESIAN_POINT ( 'NONE',  ( 133.9714219172562650, 80.45434506795683660, -2.000000000000001776 ) ) ;
#4447=DIRECTION ( 'NONE',  ( 5.551115123125772841E-17, -1.848892746611743135E-31, -1.000000000000000000 ) ) ;
#4456=CYLINDRICAL_SURFACE ( 'NONE', #3195, 5.250000000000018652 ) ;
#4457=EDGE_CURVE ( 'NONE', #1678, #484, #4768, .T. ) ;
#4462=EDGE_LOOP ( 'NONE', ( #1961, #4888, #3883 ) ) ;
#4464=ADVANCED_FACE ( 'NONE', ( #2760 ), #5279, .F. ) ;
#4465=VERTEX_POINT ( 'NONE', #1934 ) ;
#4467=CARTESIAN_POINT ( 'NONE',  ( -80.02857808274418971, -21.54565493204321669, -2.000000000000001776 ) ) ;
#4468=DIRECTION ( 'NONE',  ( -3.125627884642856345E-17, 1.000000000000000000, 1.602373713730180668E-31 ) ) ;
#4469=DIRECTION ( 'NONE',  ( -1.000000000000000000, 3.759415251443877379E-31, -5.551115123125772841E-17 ) ) ;
#4473=FACE_OUTER_BOUND ( 'NONE', #4018, .T. ) ;
#4475=DIRECTION ( 'NONE',  ( 1.000000000000000000, -3.759415251443877379E-31, 5.551115123125772841E-17 ) ) ;
#4480=CARTESIAN_POINT ( 'NONE',  ( 137.9714219172562366, -25.54565493204319182, -5.551115123125782702E-14 ) ) ;
#4481=ORIENTED_EDGE ( 'NONE', *, *, #3430, .T. ) ;
#4488=VERTEX_POINT ( 'NONE', #780 ) ;
#4489=EDGE_LOOP ( 'NONE', ( #238, #4147 ) ) ;
#4490=DIRECTION ( 'NONE',  ( 5.551115123125772841E-17, -1.848892746611743135E-31, -1.000000000000000000 ) ) ;
#4491=CARTESIAN_POINT ( 'NONE',  ( 135.7157751673381085, 75.50260479418143689, -11.99999999999995559 ) ) ;
#4499=VECTOR ( 'NONE', #1907, 1000.000000000000000 ) ;
#4500=AXIS2_PLACEMENT_3D ( 'NONE', #502, #5140, #1385 ) ;
#4501=DIRECTION ( 'NONE',  ( -0.9072577839912278064, 0.4205749795070158892, 5.551115123125773458E-17 ) ) ;
#4506=CIRCLE ( 'NONE', #2840, 5.250000000000004441 ) ;
#4510=ORIENTED_EDGE ( 'NONE', *, *, #61, .F. ) ;
#4514=ORIENTED_EDGE ( 'NONE', *, *, #1392, .T. ) ;
#4517=AXIS2_PLACEMENT_3D ( 'NONE', #5371, #698, #2412 ) ;
#4519=VERTEX_POINT ( 'NONE', #2122 ) ;
#4521=CARTESIAN_POINT ( 'NONE',  ( -80.02857808274404761, 80.45434506795689344, -9.999999999999841904 ) ) ;
#4523=PLANE ( 'NONE',  #2916 ) ;
#4524=DIRECTION ( 'NONE',  ( 5.551115123125772841E-17, -1.848892746611743354E-31, -1.000000000000000000 ) ) ;
#4526=FACE_OUTER_BOUND ( 'NONE', #2927, .T. ) ;
#4528=VERTEX_POINT ( 'NONE', #3726 ) ;
#4532=PLANE ( 'NONE',  #3217 ) ;
#4534=ADVANCED_FACE ( 'NONE', ( #5395 ), #4246, .F. ) ;
#4535=CARTESIAN_POINT ( 'NONE',  ( -82.68018911681710392, 75.92317977368848858, -9.999999999999953815 ) ) ;
#4536=ADVANCED_FACE ( 'NONE', ( #4577 ), #5056, .T. ) ;
#4538=DIRECTION ( 'NONE',  ( -1.000000000000000000, 3.759415251443877379E-31, -5.551115123125772841E-17 ) ) ;
#4541=ORIENTED_EDGE ( 'NONE', *, *, #3331, .T. ) ;
#4548=ORIENTED_EDGE ( 'NONE', *, *, #1663, .T. ) ;
#4550=CARTESIAN_POINT ( 'NONE',  ( 151.9714219172562650, -25.54565493204307813, -11.99999999999995559 ) ) ;
#4553=DIRECTION ( 'NONE',  ( 1.000000000000000000, 0.000000000000000000, 0.000000000000000000 ) ) ;
#4554=CLOSED_SHELL ( 'NONE', ( #4322, #2743, #1864, #3233, #2370, #585, #396, #3667, #4429, #3597, #1938, #4536, #5018, #2988, #3301, #4629, #2295, #2188, #2998, #4464, #1131, #3089, #3159, #258, #4187, #813, #3022, #2604, #3153, #2373, #681, #3916, #5019, #866, #2834, #2894, #230, #4293, #227, #2448, #1300, #624, #3560, #4032, #3799, #2908, #4364, #4534, #2134, #461 ) ) ;
#4561=DIRECTION ( 'NONE',  ( 1.000000000000000000, 0.000000000000000000, 7.228014483236656373E-17 ) ) ;
#4562=CARTESIAN_POINT ( 'NONE',  ( -84.02857808274407603, 84.45434506795682239, -11.99999999999995559 ) ) ;
#4569=EDGE_LOOP ( 'NONE', ( #2168, #2011, #974, #3438 ) ) ;
#4570=LINE ( 'NONE', #388, #363 ) ;
#4572=EDGE_CURVE ( 'NONE', #2971, #2111, #4506, .T. ) ;
#4573=ORIENTED_EDGE ( 'NONE', *, *, #1301, .T. ) ;
#4577=FACE_OUTER_BOUND ( 'NONE', #3673, .T. ) ;
#4578=EDGE_LOOP ( 'NONE', ( #3212, #508 ) ) ;
#4581=CARTESIAN_POINT ( 'NONE',  ( 137.9714219172562935, -25.54565493204318116, 152.0000000000004263 ) ) ;
#4584=DIRECTION ( 'NONE',  ( -1.000000000000000000, 0.000000000000000000, -8.260587980841909197E-17 ) ) ;
#4588=CARTESIAN_POINT ( 'NONE',  ( 127.9714219172562508, 80.45434506795683660, -2.000000000000002220 ) ) ;
#4591=AXIS2_PLACEMENT_3D ( 'NONE', #4480, #5296, #1539 ) ;
#4592=LINE ( 'NONE', #1625, #3670 ) ;
#4594=EDGE_CURVE ( 'NONE', #1676, #4953, #2666, .T. ) ;
#4595=EDGE_LOOP ( 'NONE', ( #1723, #1505, #5145, #2243 ) ) ;
#4596=EDGE_LOOP ( 'NONE', ( #3317, #1567, #4026, #4573 ) ) ;
#4598=AXIS2_PLACEMENT_3D ( 'NONE', #918, #505, #4788 ) ;
#4600=DIRECTION ( 'NONE',  ( -1.261617073437686134E-16, 1.000000000000000000, 1.232595164407830946E-31 ) ) ;
#4601=DIRECTION ( 'NONE',  ( 5.551115123125772841E-17, -1.848892746611743135E-31, -1.000000000000000000 ) ) ;
#4603=AXIS2_PLACEMENT_3D ( 'NONE', #4368, #595, #1453 ) ;
#4606=ORIENTED_EDGE ( 'NONE', *, *, #3189, .T. ) ;
#4607=CARTESIAN_POINT ( 'NONE',  ( 139.9714219172562366, -21.54565493204319182, -2.000000000000001332 ) ) ;
#4615=DIRECTION ( 'NONE',  ( -5.551115123125772841E-17, 1.848892746611743135E-31, 1.000000000000000000 ) ) ;
#4619=( NAMED_UNIT ( * ) SI_UNIT ( $, .STERADIAN. ) SOLID_ANGLE_UNIT ( ) );
#4623=EDGE_CURVE ( 'NONE', #979, #664, #4193, .T. ) ;
#4624=CARTESIAN_POINT ( 'NONE',  ( -74.02857808274399076, 80.45434506795689344, -2.000000000000112355 ) ) ;
#4625=DIRECTION ( 'NONE',  ( -1.000000000000000000, 0.000000000000000000, 0.000000000000000000 ) ) ;
#4629=ADVANCED_FACE ( 'NONE', ( #5031 ), #2541, .F. ) ;
#4630=EDGE_CURVE ( 'NONE', #1486, #4465, #2646, .T. ) ;
#4635=CIRCLE ( 'NONE', #2965, 5.250000000000018652 ) ;
#4645=DIRECTION ( 'NONE',  ( 1.000000000000000000, -3.759415251443877817E-31, 5.551115123125772841E-17 ) ) ;
#4646=CARTESIAN_POINT ( 'NONE',  ( 0.000000000000000000, 0.000000000000000000, 0.000000000000000000 ) ) ;
#4648=ORIENTED_EDGE ( 'NONE', *, *, #4594, .T. ) ;
#4651=CARTESIAN_POINT ( 'NONE',  ( -98.02857808274411866, 84.45434506795672291, 5.551115123125782702E-14 ) ) ;
#4653=CARTESIAN_POINT ( 'NONE',  ( -80.02857808274410445, -21.54565493204320248, -12.00000000000001066 ) ) ;
#4657=VERTEX_POINT ( 'NONE', #89 ) ;
#4658=ORIENTED_EDGE ( 'NONE', *, *, #2933, .F. ) ;
#4659=CARTESIAN_POINT ( 'NONE',  ( 128.7214219172562082, -21.54565493204319182, -2.000000000000002220 ) ) ;
#4661=PLANE ( 'NONE',  #2321 ) ;
#4663=EDGE_LOOP ( 'NONE', ( #312, #5412, #67, #2125 ) ) ;
#4666=DIRECTION ( 'NONE',  ( -1.000000000000000000, 3.759415251443877379E-31, -5.551115123125772841E-17 ) ) ;
#4672=LINE ( 'NONE', #909, #3814 ) ;
#4676=LINE ( 'NONE', #2949, #3632 ) ;
#4680=AXIS2_PLACEMENT_3D ( 'NONE', #5311, #3651, #749 ) ;
#4681=PLANE ( 'NONE',  #1245 ) ;
#4683=AXIS2_PLACEMENT_3D ( 'NONE', #893, #3864, #3518 ) ;
#4684=ORIENTED_EDGE ( 'NONE', *, *, #2685, .F. ) ;
#4688=PLANE ( 'NONE',  #805 ) ;
#4690=VECTOR ( 'NONE', #3092, 1000.000000000000000 ) ;
#4691=CIRCLE ( 'NONE', #2849, 5.250000000000018652 ) ;
#4693=ORIENTED_EDGE ( 'NONE', *, *, #3746, .F. ) ;
#4694=EDGE_CURVE ( 'NONE', #5106, #467, #2600, .T. ) ;
#4701=EDGE_CURVE ( 'NONE', #864, #2228, #301, .T. ) ;
#4703=EDGE_CURVE ( 'NONE', #3390, #3766, #3452, .T. ) ;
#4707=CARTESIAN_POINT ( 'NONE',  ( -77.37696704867103392, -26.07682022631158247, -10.00000000000000888 ) ) ;
#4708=VERTEX_POINT ( 'NONE', #4714 ) ;
#4710=VERTEX_POINT ( 'NONE', #116 ) ;
#4711=DIRECTION ( 'NONE',  ( -1.000000000000000000, 3.759415251443877379E-31, -5.551115123125772841E-17 ) ) ;
#4714=CARTESIAN_POINT ( 'NONE',  ( 139.2214219172562650, 80.45434506795679397, -12.00000000000001066 ) ) ;
#4717=EDGE_CURVE ( 'NONE', #1607, #2627, #2056, .T. ) ;
#4718=VERTEX_POINT ( 'NONE', #4738 ) ;
#4720=DIRECTION ( 'NONE',  ( 5.551115123125772841E-17, -1.848892746611743135E-31, -1.000000000000000000 ) ) ;
#4723=ORIENTED_EDGE ( 'NONE', *, *, #499, .T. ) ;
#4727=DIRECTION ( 'NONE',  ( 0.9072577839912278064, -0.4205749795070158892, -5.551115123125773458E-17 ) ) ;
#4737=FACE_OUTER_BOUND ( 'NONE', #4596, .T. ) ;
#4738=CARTESIAN_POINT ( 'NONE',  ( -81.77293133282597637, -16.59391465826784540, -10.00000000000000888 ) ) ;
#4743=LINE ( 'NONE', #1881, #544 ) ;
#4746=EDGE_LOOP ( 'NONE', ( #3641, #3836, #4295, #5094, #4789, #3829, #4693, #4002 ) ) ;
#4752=ORIENTED_EDGE ( 'NONE', *, *, #5189, .T. ) ;
#4754=ORIENTED_EDGE ( 'NONE', *, *, #3479, .F. ) ;
#4755=CIRCLE ( 'NONE', #2040, 14.00000000000001243 ) ;
#4758=DIRECTION ( 'NONE',  ( -1.000000000000000000, 0.000000000000000000, 0.000000000000000000 ) ) ;
#4759=AXIS2_PLACEMENT_3D ( 'NONE', #5030, #4601, #1271 ) ;
#4763=CIRCLE ( 'NONE', #4500, 6.000000000000032863 ) ;
#4768=CIRCLE ( 'NONE', #1785, 5.250000000000004441 ) ;
#4779=ORIENTED_EDGE ( 'NONE', *, *, #3563, .T. ) ;
#4780=EDGE_CURVE ( 'NONE', #556, #1493, #4080, .T. ) ;
#4786=ORIENTED_EDGE ( 'NONE', *, *, #3974, .T. ) ;
#4788=DIRECTION ( 'NONE',  ( 1.000000000000000000, 0.000000000000000000, 0.000000000000000000 ) ) ;
#4789=ORIENTED_EDGE ( 'NONE', *, *, #1972, .F. ) ;
#4798=ORIENTED_EDGE ( 'NONE', *, *, #1211, .T. ) ;
#4803=ORIENTED_EDGE ( 'NONE', *, *, #2679, .F. ) ;
#4807=EDGE_LOOP ( 'NONE', ( #52, #2284, #806 ) ) ;
#4808=DIRECTION ( 'NONE',  ( -5.551115123125772841E-17, 1.848892746611743135E-31, 1.000000000000000000 ) ) ;
#4810=ORIENTED_EDGE ( 'NONE', *, *, #4572, .F. ) ;
#4811=ORIENTED_EDGE ( 'NONE', *, *, #4363, .F. ) ;
#4819=DIRECTION ( 'NONE',  ( 5.551115123125772841E-17, -1.848892746611743135E-31, -1.000000000000000000 ) ) ;
#4820=CARTESIAN_POINT ( 'NONE',  ( 139.9714219172562650, -21.54565493204319182, -12.00000000000006573 ) ) ;
#4822=DIRECTION ( 'NONE',  ( 1.000000000000000000, 0.000000000000000000, 8.260587980841909197E-17 ) ) ;
#4823=EDGE_CURVE ( 'NONE', #4034, #4718, #5386, .T. ) ;
#4832=DIRECTION ( 'NONE',  ( 0.4205749795070160557, -0.9072577839912276954, -5.551115123125780853E-17 ) ) ;
#4834=ORIENTED_EDGE ( 'NONE', *, *, #4701, .F. ) ;
#4835=ORIENTED_EDGE ( 'NONE', *, *, #3318, .F. ) ;
#4841=DIRECTION ( 'NONE',  ( -5.551115123125772841E-17, 1.848892746611743135E-31, 1.000000000000000000 ) ) ;
#4843=CIRCLE ( 'NONE', #4759, 5.250000000000018652 ) ;
#4844=( NAMED_UNIT ( * ) PLANE_ANGLE_UNIT ( ) SI_UNIT ( $, .RADIAN. ) );
#4846=CARTESIAN_POINT ( 'NONE',  ( -80.02857808274418971, -21.54565493204321669, -2.000000000000001776 ) ) ;
#4847=CARTESIAN_POINT ( 'NONE',  ( 127.9714219172562224, 80.45434506795683660, -12.00000000000001066 ) ) ;
#4848=CARTESIAN_POINT ( 'NONE',  ( -80.02857808274401918, 80.45434506795689344, -2.000000000000112799 ) ) ;
#4849=CIRCLE ( 'NONE', #4591, 14.00000000000001243 ) ;
#4850=AXIS2_PLACEMENT_3D ( 'NONE', #5339, #3238, #716 ) ;
#4851=LINE ( 'NONE', #1091, #4416 ) ;
#4854=VECTOR ( 'NONE', #4007, 1000.000000000000000 ) ;
#4856=DIRECTION ( 'NONE',  ( 5.551115123125772841E-17, -1.848892746611743135E-31, -1.000000000000000000 ) ) ;
#4861=VECTOR ( 'NONE', #2283, 1000.000000000000000 ) ;
#4863=VECTOR ( 'NONE', #4615, 1000.000000000000000 ) ;
#4866=ORIENTED_EDGE ( 'NONE', *, *, #3721, .F. ) ;
#4867=VECTOR ( 'NONE', #3305, 1000.000000000000000 ) ;
#4870=CARTESIAN_POINT ( 'NONE',  ( -77.37696704867106234, 84.98551036222526989, -9.999999999999953815 ) ) ;
#4871=VERTEX_POINT ( 'NONE', #4870 ) ;
#4876=DIRECTION ( 'NONE',  ( -5.551115123125772841E-17, 1.848892746611743135E-31, 1.000000000000000000 ) ) ;
#4879=PLANE ( 'NONE',  #2667 ) ;
#4881=CARTESIAN_POINT ( 'NONE',  ( -84.02857808274418971, -25.54565493204318116, -5.551115123125782702E-14 ) ) ;
#4882=DIRECTION ( 'NONE',  ( -0.4205749795070160557, 0.9072577839912276954, 5.551115123125780853E-17 ) ) ;
#4888=ORIENTED_EDGE ( 'NONE', *, *, #1972, .T. ) ;
#4894=ORIENTED_EDGE ( 'NONE', *, *, #1036, .F. ) ;
#4896=ORIENTED_EDGE ( 'NONE', *, *, #1284, .F. ) ;
#4897=DIRECTION ( 'NONE',  ( -1.000000000000000000, 0.000000000000000000, 0.000000000000000000 ) ) ;
#4899=CARTESIAN_POINT ( 'NONE',  ( 133.9714219172562366, -21.54565493204319182, -26.84924240491753977 ) ) ;
#4902=CARTESIAN_POINT ( 'NONE',  ( 136.6230329513292645, -17.01448963777482248, -12.00000000000001066 ) ) ;
#4903=DIRECTION ( 'NONE',  ( -0.9072577839912275843, -0.4205749795070160002, -1.110223024625155801E-16 ) ) ;
#4907=CYLINDRICAL_SURFACE ( 'NONE', #1252, 14.00000000000002665 ) ;
#4914=ORIENTED_EDGE ( 'NONE', *, *, #1664, .T. ) ;
#4921=EDGE_CURVE ( 'NONE', #4871, #4528, #710, .T. ) ;
#4924=EDGE_CURVE ( 'NONE', #4718, #1930, #3644, .T. ) ;
#4928=ORIENTED_EDGE ( 'NONE', *, *, #4363, .T. ) ;
#4929=CIRCLE ( 'NONE', #3877, 5.250000000000004441 ) ;
#4930=( LENGTH_UNIT ( ) NAMED_UNIT ( * ) SI_UNIT ( .MILLI., .METRE. ) );
#4933=DIRECTION ( 'NONE',  ( 5.551115123125772841E-17, -1.848892746611743354E-31, -1.000000000000000000 ) ) ;
#4937=CARTESIAN_POINT ( 'NONE',  ( 133.9714219172562650, 80.45434506795683660, -2.000000000000001776 ) ) ;
#4943=AXIS2_PLACEMENT_3D ( 'NONE', #609, #1397, #5199 ) ;
#4945=ORIENTED_EDGE ( 'NONE', *, *, #2999, .T. ) ;
#4947=EDGE_LOOP ( 'NONE', ( #4684, #2178 ) ) ;
#4948=ADVANCED_FACE ( 'NONE', ( #3235 ), #2752, .F. ) ;
#4952=FACE_OUTER_BOUND ( 'NONE', #3000, .T. ) ;
#4953=VERTEX_POINT ( 'NONE', #364 ) ;
#4957=CARTESIAN_POINT ( 'NONE',  ( -98.02857808274420393, -25.54565493204309234, 5.551115123125782702E-14 ) ) ;
#4960=PLANE ( 'NONE',  #2138 ) ;
#4961=AXIS2_PLACEMENT_3D ( 'NONE', #2247, #3154, #2684 ) ;
#4963=CARTESIAN_POINT ( 'NONE',  ( -84.02857808274397655, 98.45434506795682239, 152.0000000000000853 ) ) ;
#4964=ORIENTED_EDGE ( 'NONE', *, *, #490, .F. ) ;
#4965=ORIENTED_EDGE ( 'NONE', *, *, #2078, .F. ) ;
#4968=CARTESIAN_POINT ( 'NONE',  ( -84.02857808274397655, 98.45434506795682239, 152.0000000000000853 ) ) ;
#4969=CYLINDRICAL_SURFACE ( 'NONE', #3024, 6.000000000000032863 ) ;
#4970=PLANE ( 'NONE',  #2357 ) ;
#4974=ORIENTED_EDGE ( 'NONE', *, *, #617, .F. ) ;
#4975=CARTESIAN_POINT ( 'NONE',  ( -84.02857808274413287, 84.45434506795682239, -5.551115123125782702E-14 ) ) ;
#4978=ORIENTED_EDGE ( 'NONE', *, *, #4703, .F. ) ;
#4980=LINE ( 'NONE', #5029, #2553 ) ;
#4981=DIRECTION ( 'NONE',  ( -1.000000000000000000, 0.000000000000000000, 0.000000000000000000 ) ) ;
#4984=ORIENTED_EDGE ( 'NONE', *, *, #5228, .T. ) ;
#4986=CARTESIAN_POINT ( 'NONE',  ( -80.02857808274401918, 80.45434506795689344, -2.000000000000112799 ) ) ;
#4987=DIRECTION ( 'NONE',  ( 5.551115123125772841E-17, -1.848892746611743354E-31, -1.000000000000000000 ) ) ;
#4995=VERTEX_POINT ( 'NONE', #1291 ) ;
#5001=FACE_OUTER_BOUND ( 'NONE', #3775, .T. ) ;
#5005=ORIENTED_EDGE ( 'NONE', *, *, #2078, .T. ) ;
#5008=DIRECTION ( 'NONE',  ( -1.000000000000000000, 3.759415251443877379E-31, -5.551115123125772841E-17 ) ) ;
#5010=AXIS2_PLACEMENT_3D ( 'NONE', #2287, #4720, #1469 ) ;
#5013=CARTESIAN_POINT ( 'NONE',  ( 137.9714219172563219, 84.45434506795683660, 152.0000000000003126 ) ) ;
#5018=ADVANCED_FACE ( 'NONE', ( #4952 ), #1626, .T. ) ;
#5019=ADVANCED_FACE ( 'NONE', ( #2510 ), #878, .T. ) ;
#5022=DIRECTION ( 'NONE',  ( -3.204747427460360459E-31, 1.000000000000000000, -1.848892746611743354E-31 ) ) ;
#5023=CIRCLE ( 'NONE', #5288, 5.250000000000018652 ) ;
#5024=VERTEX_POINT ( 'NONE', #3748 ) ;
#5029=CARTESIAN_POINT ( 'NONE',  ( -98.02857808274411866, 84.45434506795672291, -12.00000000000001066 ) ) ;
#5030=CARTESIAN_POINT ( 'NONE',  ( -80.02857808274410445, -21.54565493204320248, -12.00000000000001066 ) ) ;
#5031=FACE_OUTER_BOUND ( 'NONE', #447, .T. ) ;
#5033=AXIS2_PLACEMENT_3D ( 'NONE', #77, #2993, #4666 ) ;
#5036=ORIENTED_EDGE ( 'NONE', *, *, #3394, .F. ) ;
#5044=DIRECTION ( 'NONE',  ( 1.000000000000000000, 0.000000000000000000, 0.000000000000000000 ) ) ;
#5045=ORIENTED_EDGE ( 'NONE', *, *, #1083, .F. ) ;
#5046=EDGE_CURVE ( 'NONE', #5400, #1486, #739, .T. ) ;
#5047=EDGE_LOOP ( 'NONE', ( #962, #569, #2453, #4752 ) ) ;
#5051=LINE ( 'NONE', #721, #3648 ) ;
#5055=FACE_OUTER_BOUND ( 'NONE', #5118, .T. ) ;
#5056=PLANE ( 'NONE',  #1873 ) ;
#5057=VECTOR ( 'NONE', #571, 1000.000000000000000 ) ;
#5059=ORIENTED_EDGE ( 'NONE', *, *, #1664, .F. ) ;
#5063=AXIS2_PLACEMENT_3D ( 'NONE', #3934, #986, #619 ) ;
#5064=CARTESIAN_POINT ( 'NONE',  ( -84.02857808274407603, 84.45434506795682239, -11.99999999999995559 ) ) ;
#5065=DIRECTION ( 'NONE',  ( -5.551115123125772841E-17, 1.848892746611743135E-31, 1.000000000000000000 ) ) ;
#5066=CARTESIAN_POINT ( 'NONE',  ( 133.9714219172562366, -21.54565493204319182, -2.000000000000001776 ) ) ;
#5067=ORIENTED_EDGE ( 'NONE', *, *, #1060, .F. ) ;
#5080=CARTESIAN_POINT ( 'NONE',  ( 133.9714219172562366, -21.54565493204319182, -2.000000000000001776 ) ) ;
#5082=VECTOR ( 'NONE', #3361, 1000.000000000000114 ) ;
#5084=ORIENTED_EDGE ( 'NONE', *, *, #5283, .T. ) ;
#5085=EDGE_CURVE ( 'NONE', #1327, #4236, #4672, .T. ) ;
#5090=DIRECTION ( 'NONE',  ( -5.551115123125772841E-17, 1.848892746611743135E-31, 1.000000000000000000 ) ) ;
#5093=DIRECTION ( 'NONE',  ( -1.000000000000000000, 0.000000000000000000, -7.228014483236656373E-17 ) ) ;
#5094=ORIENTED_EDGE ( 'NONE', *, *, #3687, .F. ) ;
#5097=DIRECTION ( 'NONE',  ( -1.000000000000000000, 0.000000000000000000, 0.000000000000000000 ) ) ;
#5100=EDGE_LOOP ( 'NONE', ( #945, #2345 ) ) ;
#5101=LINE ( 'NONE', #4707, #509 ) ;
#5102=( LENGTH_UNIT ( ) NAMED_UNIT ( * ) SI_UNIT ( .MILLI., .METRE. ) );
#5103=EDGE_CURVE ( 'NONE', #783, #1799, #3645, .T. ) ;
#5105=EDGE_CURVE ( 'NONE', #3075, #467, #3019, .T. ) ;
#5106=VERTEX_POINT ( 'NONE', #3568 ) ;
#5111=CIRCLE ( 'NONE', #380, 6.000000000000032863 ) ;
#5113=LINE ( 'NONE', #3065, #3363 ) ;
#5114=DIRECTION ( 'NONE',  ( 5.551115123125772841E-17, -1.848892746611743135E-31, -1.000000000000000000 ) ) ;
#5117=ORIENTED_EDGE ( 'NONE', *, *, #3117, .F. ) ;
#5118=EDGE_LOOP ( 'NONE', ( #1098, #579, #3813, #1276 ) ) ;
#5123=EDGE_CURVE ( 'NONE', #864, #1607, #3618, .T. ) ;
#5124=VECTOR ( 'NONE', #473, 1000.000000000000000 ) ;
#5125=FACE_OUTER_BOUND ( 'NONE', #1675, .T. ) ;
#5126=EDGE_LOOP ( 'NONE', ( #1740, #1869, #4974, #3786 ) ) ;
#5132=LINE ( 'NONE', #650, #1797 ) ;
#5133=APPLICATION_CONTEXT ( 'automotive_design' ) ;
#5135=DIRECTION ( 'NONE',  ( 5.551115123125772841E-17, -1.848892746611743135E-31, -1.000000000000000000 ) ) ;
#5136=LINE ( 'NONE', #3031, #2088 ) ;
#5140=DIRECTION ( 'NONE',  ( 5.551115123125772841E-17, -1.848892746611743135E-31, -1.000000000000000000 ) ) ;
#5143=CARTESIAN_POINT ( 'NONE',  ( 139.9714219172562650, -21.54565493204319182, -2.000000000000001332 ) ) ;
#5144=CARTESIAN_POINT ( 'NONE',  ( 137.9714219172561229, -39.54565493204319182, 152.0000000000004263 ) ) ;
#5145=ORIENTED_EDGE ( 'NONE', *, *, #2585, .F. ) ;
#5147=VERTEX_POINT ( 'NONE', #317 ) ;
#5152=ORIENTED_EDGE ( 'NONE', *, *, #2944, .T. ) ;
#5153=AXIS2_PLACEMENT_3D ( 'NONE', #2612, #1855, #3542 ) ;
#5158=EDGE_CURVE ( 'NONE', #1066, #4519, #5378, .T. ) ;
#5162=EDGE_CURVE ( 'NONE', #467, #4218, #3592, .T. ) ;
#5167=CARTESIAN_POINT ( 'NONE',  ( 139.2214219172562650, -21.54565493204319182, -12.00000000000006573 ) ) ;
#5168=DIRECTION ( 'NONE',  ( -1.000000000000000000, 0.000000000000000000, -5.551115123125777155E-17 ) ) ;
#5169=EDGE_LOOP ( 'NONE', ( #3030, #3029 ) ) ;
#5173=DIRECTION ( 'NONE',  ( 5.551115123125772841E-17, -1.848892746611743135E-31, -1.000000000000000000 ) ) ;
#5177=ORIENTED_EDGE ( 'NONE', *, *, #3887, .F. ) ;
#5180=CARTESIAN_POINT ( 'NONE',  ( 137.9714219172561798, -39.54565493204318471, -5.551115123125782702E-14 ) ) ;
#5183=PRODUCT_CONTEXT ( 'NONE', #5133, 'mechanical' ) ;
#5184=EDGE_CURVE ( 'NONE', #179, #1676, #2403, .T. ) ;
#5185=ORIENTED_EDGE ( 'NONE', *, *, #4694, .F. ) ;
#5187=ORIENTED_EDGE ( 'NONE', *, *, #3507, .T. ) ;
#5189=EDGE_CURVE ( 'NONE', #1486, #2971, #4003, .T. ) ;
#5193=ORIENTED_EDGE ( 'NONE', *, *, #5330, .T. ) ;
#5195=CIRCLE ( 'NONE', #5289, 5.250000000000018652 ) ;
#5197=CARTESIAN_POINT ( 'NONE',  ( -78.28422483266231779, -26.49739520581859153, -10.00000000000006395 ) ) ;
#5199=DIRECTION ( 'NONE',  ( -1.000000000000000000, 0.000000000000000000, -7.228014483236656373E-17 ) ) ;
#5202=AXIS2_PLACEMENT_3D ( 'NONE', #1584, #3308, #329 ) ;
#5203=( LENGTH_UNIT ( ) NAMED_UNIT ( * ) SI_UNIT ( .MILLI., .METRE. ) );
#5210=DIRECTION ( 'NONE',  ( -0.9072577839912278064, 0.4205749795070158892, 5.551115123125773458E-17 ) ) ;
#5217=ORIENTED_EDGE ( 'NONE', *, *, #1736, .F. ) ;
#5219=EDGE_CURVE ( 'NONE', #3515, #3069, #2838, .T. ) ;
#5221=CARTESIAN_POINT ( 'NONE',  ( -80.02857808274410445, -21.54565493204320248, -26.84924240491759662 ) ) ;
#5222=DIRECTION ( 'NONE',  ( 1.000000000000000000, 0.000000000000000000, 0.000000000000000000 ) ) ;
#5225=ORIENTED_EDGE ( 'NONE', *, *, #1436, .F. ) ;
#5227=CARTESIAN_POINT ( 'NONE',  ( -80.02857808274410445, -21.54565493204321669, -9.999999999999953815 ) ) ;
#5228=EDGE_CURVE ( 'NONE', #2780, #1607, #260, .T. ) ;
#5230=PLANE ( 'NONE',  #4961 ) ;
#5231=DIRECTION ( 'NONE',  ( 1.000000000000000000, 0.000000000000000000, 0.000000000000000000 ) ) ;
#5235=DIRECTION ( 'NONE',  ( -5.551115123125772841E-17, 1.848892746611743135E-31, 1.000000000000000000 ) ) ;
#5236=CARTESIAN_POINT ( 'NONE',  ( -80.02857808274401918, 80.45434506795689344, -12.00000000000001066 ) ) ;
#5245=DIRECTION ( 'NONE',  ( 5.551115123125772841E-17, -1.848892746611743135E-31, -1.000000000000000000 ) ) ;
#5247=ORIENTED_EDGE ( 'NONE', *, *, #4630, .F. ) ;
#5250=DIRECTION ( 'NONE',  ( 5.551115123125772841E-17, -1.848892746611743135E-31, -1.000000000000000000 ) ) ;
#5251=CARTESIAN_POINT ( 'NONE',  ( 136.6230329513292361, -17.01448963777488288, -9.999999999999953815 ) ) ;
#5252=DIRECTION ( 'NONE',  ( 5.551115123125772841E-17, -1.848892746611743354E-31, -1.000000000000000000 ) ) ;
#5254=LINE ( 'NONE', #3156, #1177 ) ;
#5255=ORIENTED_EDGE ( 'NONE', *, *, #3631, .T. ) ;
#5259=EDGE_CURVE ( 'NONE', #179, #534, #3375, .T. ) ;
#5267=ORIENTED_EDGE ( 'NONE', *, *, #1604, .F. ) ;
#5273=ORIENTED_EDGE ( 'NONE', *, *, #4229, .F. ) ;
#5275=DIRECTION ( 'NONE',  ( 5.551115123125772841E-17, -1.848892746611743135E-31, -1.000000000000000000 ) ) ;
#5276=AXIS2_PLACEMENT_3D ( 'NONE', #1933, #4468, #4030 ) ;
#5277=DIRECTION ( 'NONE',  ( 1.000000000000000000, 0.000000000000000000, 0.000000000000000000 ) ) ;
#5279=PLANE ( 'NONE',  #3107 ) ;
#5280=( NAMED_UNIT ( * ) SI_UNIT ( $, .STERADIAN. ) SOLID_ANGLE_UNIT ( ) );
#5283=EDGE_CURVE ( 'NONE', #1569, #994, #5195, .T. ) ;
#5284=DIRECTION ( 'NONE',  ( -1.000000000000000000, 3.759415251443877379E-31, -5.551115123125772841E-17 ) ) ;
#5288=AXIS2_PLACEMENT_3D ( 'NONE', #5236, #2691, #2329 ) ;
#5289=AXIS2_PLACEMENT_3D ( 'NONE', #1218, #3751, #3343 ) ;
#5290=DIRECTION ( 'NONE',  ( -5.551115123125772841E-17, 1.848892746611743135E-31, 1.000000000000000000 ) ) ;
#5292=VECTOR ( 'NONE', #3658, 1000.000000000000000 ) ;
#5293=CYLINDRICAL_SURFACE ( 'NONE', #252, 5.250000000000004441 ) ;
#5296=DIRECTION ( 'NONE',  ( -5.551115123125772841E-17, 1.848892746611743135E-31, 1.000000000000000000 ) ) ;
#5297=AXIS2_PLACEMENT_3D ( 'NONE', #2091, #4238, #3768 ) ;
#5305=DIRECTION ( 'NONE',  ( 5.551115123125772841E-17, -1.848892746611743135E-31, -1.000000000000000000 ) ) ;
#5306=CARTESIAN_POINT ( 'NONE',  ( -81.77293133282597637, -16.59391465826784540, -10.00000000000000888 ) ) ;
#5307=EDGE_LOOP ( 'NONE', ( #2535, #4008 ) ) ;
#5311=CARTESIAN_POINT ( 'NONE',  ( 137.9714219172562650, 84.45434506795687923, -5.551115123125782702E-14 ) ) ;
#5314=DIRECTION ( 'NONE',  ( -1.000000000000000000, 3.759415251443877379E-31, -5.551115123125772841E-17 ) ) ;
#5315=DIRECTION ( 'NONE',  ( 5.551115123125772841E-17, -1.848892746611743135E-31, -1.000000000000000000 ) ) ;
#5321=FACE_OUTER_BOUND ( 'NONE', #3622, .T. ) ;
#5322=DIRECTION ( 'NONE',  ( -5.551115123125772841E-17, 1.848892746611743354E-31, 1.000000000000000000 ) ) ;
#5328=ADVANCED_FACE ( 'NONE', ( #5001 ), #3697, .T. ) ;
#5330=EDGE_CURVE ( 'NONE', #2627, #4404, #2537, .T. ) ;
#5333=EDGE_CURVE ( 'NONE', #1369, #5147, #856, .T. ) ;
#5336=ORIENTED_EDGE ( 'NONE', *, *, #2519, .F. ) ;
#5339=CARTESIAN_POINT ( 'NONE',  ( -80.02857808274418971, -21.54565493204321669, -2.000000000000001776 ) ) ;
#5344=LINE ( 'NONE', #440, #1616 ) ;
#5346=CARTESIAN_POINT ( 'NONE',  ( 133.9714219172562366, -21.54565493204323090, -9.999999999999841904 ) ) ;
#5347=CARTESIAN_POINT ( 'NONE',  ( -85.27857808274410445, -21.54565493204320248, -12.00000000000001066 ) ) ;
#5348=CARTESIAN_POINT ( 'NONE',  ( 151.9714219172562650, -25.54565493204307813, -11.99999999999995559 ) ) ;
#5351=CARTESIAN_POINT ( 'NONE',  ( 133.9714219172562366, -21.54565493204319182, -2.000000000000001776 ) ) ;
#5354=ORIENTED_EDGE ( 'NONE', *, *, #5105, .F. ) ;
#5365=LINE ( 'NONE', #1194, #4499 ) ;
#5367=DIRECTION ( 'NONE',  ( -1.000000000000000000, 0.000000000000000000, 0.000000000000000000 ) ) ;
#5368=VERTEX_POINT ( 'NONE', #4957 ) ;
#5371=CARTESIAN_POINT ( 'NONE',  ( -84.02857808274413287, 84.45434506795682239, 152.0000000000003126 ) ) ;
#5378=CIRCLE ( 'NONE', #4850, 6.000000000000032863 ) ;
#5385=DIRECTION ( 'NONE',  ( 5.551115123125772841E-17, -1.848892746611743135E-31, -1.000000000000000000 ) ) ;
#5386=CIRCLE ( 'NONE', #3027, 5.250000000000018652 ) ;
#5388=ORIENTED_EDGE ( 'NONE', *, *, #2878, .T. ) ;
#5389=CIRCLE ( 'NONE', #3388, 5.250000000000031974 ) ;
#5394=DIRECTION ( 'NONE',  ( -5.551115123125772841E-17, 1.848892746611743354E-31, 1.000000000000000000 ) ) ;
#5395=FACE_OUTER_BOUND ( 'NONE', #1997, .T. ) ;
#5397=VERTEX_POINT ( 'NONE', #2513 ) ;
#5398=EDGE_CURVE ( 'NONE', #1369, #2476, #2491, .T. ) ;
#5400=VERTEX_POINT ( 'NONE', #1269 ) ;
#5402=CARTESIAN_POINT ( 'NONE',  ( -80.02857808274413287, 80.45434506795689344, -26.84924240491753977 ) ) ;
#5404=DIRECTION ( 'NONE',  ( 5.551115123125772841E-17, -1.848892746611743135E-31, -1.000000000000000000 ) ) ;
#5409=EDGE_LOOP ( 'NONE', ( #4811, #4541, #3866, #9, #2, #3405, #4810, #4514 ) ) ;
#5410=LINE ( 'NONE', #1644, #1022 ) ;
#5412=ORIENTED_EDGE ( 'NONE', *, *, #1604, .T. ) ;
#5413=EDGE_LOOP ( 'NONE', ( #2649, #874, #2889, #1550 ) ) ;
#5417=CARTESIAN_POINT ( 'NONE',  ( 133.9714219172562366, -21.54565493204319182, -2.000000000000001776 ) ) ;
#5421=ORIENTED_EDGE ( 'NONE', *, *, #2685, .T. ) ;
#5428=EDGE_CURVE ( 'NONE', #4465, #800, #1705, .T. ) ;
#5430=EDGE_CURVE ( 'NONE', #2476, #5147, #3202, .T. ) ;
#5452=COLOUR_RGB('Sky Blue',0.24,0.69,0.87);
#5453=FILL_AREA_STYLE_COLOUR('',#5452);
#5454=FILL_AREA_STYLE('',(#5453));
#5455=SURFACE_STYLE_FILL_AREA(#5454);
#5456=SURFACE_SIDE_STYLE('',(#5455));
#5457=SURFACE_STYLE_USAGE(.BOTH.,#5456);
#5458=PRESENTATION_STYLE_ASSIGNMENT((#5457));
ENDSEC;
END-ISO-10303-21;
